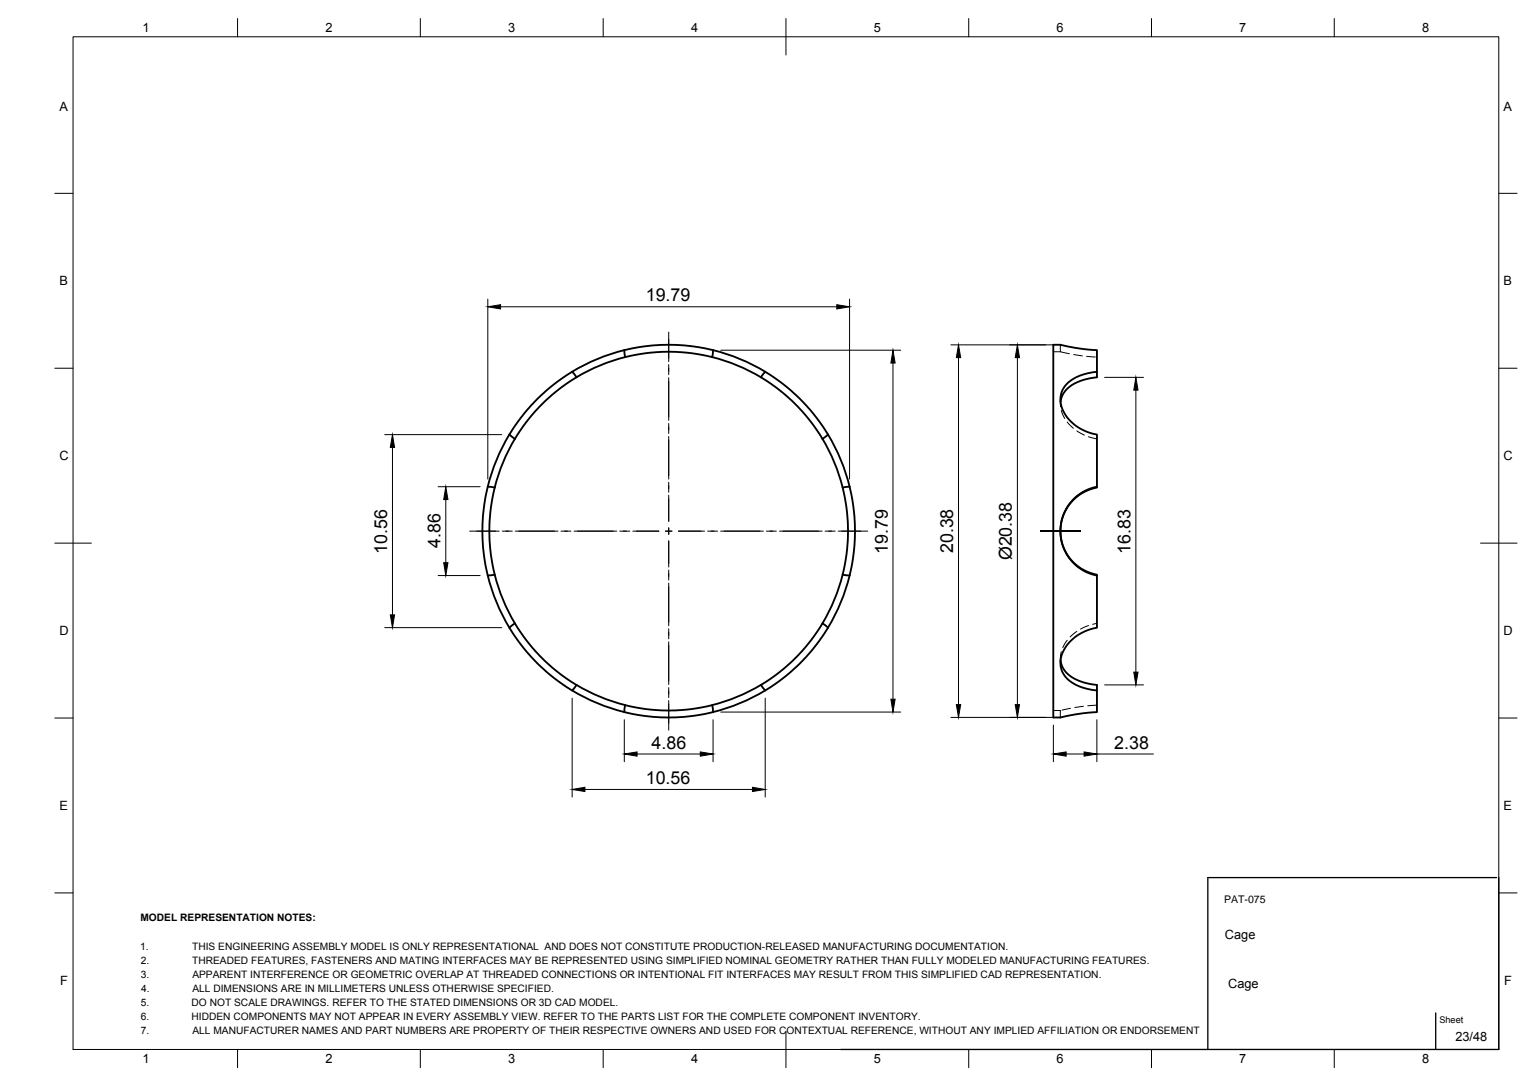
ISO-10303-21;
HEADER;
/* Generated by software containing ST-Developer
 * from STEP Tools, Inc. (www.steptools.com) 
 */

FILE_DESCRIPTION(
/* description */ ('Over-Centre Plunger Toggle Clamp on Slotted Fixture Frame'),
/* implementation_level */ '2;1');

FILE_NAME(
/* name */ 
'Cage.step',
/* time_stamp */ '2026-10-28T03:23:24-07:00',
/* author */ (''),
/* organization */ (''),
/* preprocessor_version */ 'ST-DEVELOPER v20.2',
/* originating_system */ 'Autodesk Translation Framework v15.17.0.0',
/* authorisation */ '');

FILE_SCHEMA (('AUTOMOTIVE_DESIGN { 1 0 10303 214 3 1 1 }'));
ENDSEC;

DATA;
#10=MECHANICAL_DESIGN_GEOMETRIC_PRESENTATION_REPRESENTATION('',(#539),#15212);
#355=B_SPLINE_CURVE_WITH_KNOTS('',3,(#13605,#13606,#13607,#13608,#13609,
#13610,#13611,#13612,#13613,#13614,#13615,#13616,#13617,#13618,#13619,#13620,
#13621,#13622,#13623,#13624,#13625,#13626),.UNSPECIFIED.,.F.,.F.,(4,2,2,
2,2,2,2,2,2,2,4),(0.0473477652366656,0.126350602536658,0.189525903804987,
0.252701205073317,0.313298422430275,0.373895639787233,0.434492857144191,
0.495090074501149,0.558265375769478,0.621440677037807,0.7004435143378),
 .UNSPECIFIED.);
#356=B_SPLINE_CURVE_WITH_KNOTS('',3,(#13630,#13631,#13632,#13633,#13634,
#13635,#13636,#13637,#13638,#13639,#13640,#13641,#13642,#13643,#13644,#13645,
#13646,#13647,#13648,#13649,#13650,#13651),.UNSPECIFIED.,.F.,.F.,(4,2,2,
2,2,2,2,2,2,2,4),(0.0464897534940957,0.0852567806515119,0.170513561303024,
0.246687263103517,0.308657850341199,0.370628437578881,0.432599024816563,
0.494569612054245,0.570743313854739,0.656000094506251,0.694767121663666),
 .UNSPECIFIED.);
#357=B_SPLINE_CURVE_WITH_KNOTS('',3,(#13657,#13658,#13659,#13660,#13661,
#13662,#13663,#13664,#13665,#13666,#13667,#13668,#13669,#13670,#13671,#13672,
#13673,#13674,#13675,#13676,#13677,#13678),.UNSPECIFIED.,.F.,.F.,(4,2,2,
2,2,2,2,2,2,2,4),(0.0464897534940957,0.0852567806515118,0.170513561303024,
0.246687263103517,0.308657850341199,0.370628437578881,0.432599024816563,
0.494569612054245,0.570743313854738,0.65600009450625,0.694767121663666),
 .UNSPECIFIED.);
#358=B_SPLINE_CURVE_WITH_KNOTS('',3,(#13682,#13683,#13684,#13685,#13686,
#13687,#13688,#13689,#13690,#13691,#13692,#13693,#13694,#13695,#13696,#13697,
#13698,#13699,#13700,#13701,#13702,#13703),.UNSPECIFIED.,.F.,.F.,(4,2,2,
2,2,2,2,2,2,2,4),(0.0464897534940957,0.0852567806515119,0.170513561303024,
0.246687263103517,0.308657850341199,0.370628437578881,0.432599024816563,
0.494569612054245,0.570743313854739,0.656000094506251,0.694767121663666),
 .UNSPECIFIED.);
#359=B_SPLINE_CURVE_WITH_KNOTS('',3,(#13707,#13708,#13709,#13710,#13711,
#13712,#13713,#13714,#13715,#13716,#13717,#13718),.UNSPECIFIED.,.F.,.F.,
(4,2,2,2,2,4),(0.0464897534940957,0.0852567806515119,0.170513561303024,
0.246687263103517,0.308657850341199,0.370628437578881),.UNSPECIFIED.);
#360=B_SPLINE_CURVE_WITH_KNOTS('',3,(#13723,#13724,#13725,#13726,#13727,
#13728,#13729,#13730,#13731,#13732,#13733,#13734),.UNSPECIFIED.,.F.,.F.,
(4,2,2,2,2,4),(0.370628437578881,0.432599024816563,0.494569612054245,0.570743313854738,
0.65600009450625,0.694767121663666),.UNSPECIFIED.);
#361=B_SPLINE_CURVE_WITH_KNOTS('',3,(#13738,#13739,#13740,#13741,#13742,
#13743,#13744,#13745,#13746,#13747,#13748,#13749,#13750,#13751,#13752,#13753,
#13754,#13755,#13756,#13757,#13758,#13759),.UNSPECIFIED.,.F.,.F.,(4,2,2,
2,2,2,2,2,2,2,4),(0.0464897534940957,0.0852567806515121,0.170513561303024,
0.246687263103518,0.308657850341199,0.370628437578881,0.432599024816563,
0.494569612054245,0.570743313854738,0.65600009450625,0.694767121663666),
 .UNSPECIFIED.);
#362=B_SPLINE_CURVE_WITH_KNOTS('',3,(#13763,#13764,#13765,#13766,#13767,
#13768,#13769,#13770,#13771,#13772,#13773,#13774,#13775,#13776,#13777,#13778,
#13779,#13780,#13781,#13782,#13783,#13784),.UNSPECIFIED.,.F.,.F.,(4,2,2,
2,2,2,2,2,2,2,4),(0.0464897534940957,0.0852567806515119,0.170513561303024,
0.246687263103517,0.308657850341199,0.370628437578881,0.432599024816563,
0.494569612054245,0.570743313854738,0.65600009450625,0.694767121663667),
 .UNSPECIFIED.);
#363=B_SPLINE_CURVE_WITH_KNOTS('',3,(#13788,#13789,#13790,#13791,#13792,
#13793,#13794,#13795,#13796,#13797,#13798,#13799,#13800,#13801,#13802,#13803,
#13804,#13805,#13806,#13807,#13808,#13809),.UNSPECIFIED.,.F.,.F.,(4,2,2,
2,2,2,2,2,2,2,4),(0.0464897534940957,0.0852567806515119,0.170513561303024,
0.246687263103517,0.308657850341199,0.370628437578881,0.432599024816563,
0.494569612054245,0.570743313854738,0.65600009450625,0.694767121663666),
 .UNSPECIFIED.);
#364=B_SPLINE_CURVE_WITH_KNOTS('',3,(#13813,#13814,#13815,#13816,#13817,
#13818,#13819,#13820,#13821,#13822,#13823,#13824,#13825,#13826,#13827,#13828,
#13829,#13830,#13831,#13832,#13833,#13834),.UNSPECIFIED.,.F.,.F.,(4,2,2,
2,2,2,2,2,2,2,4),(0.0464897534940957,0.0852567806515119,0.170513561303024,
0.246687263103517,0.308657850341199,0.370628437578881,0.432599024816563,
0.494569612054245,0.570743313854739,0.656000094506251,0.694767121663667),
 .UNSPECIFIED.);
#365=B_SPLINE_CURVE_WITH_KNOTS('',3,(#13842,#13843,#13844,#13845,#13846,
#13847,#13848,#13849,#13850,#13851,#13852,#13853,#13854,#13855,#13856,#13857,
#13858,#13859,#13860,#13861,#13862,#13863),.UNSPECIFIED.,.F.,.F.,(4,2,2,
2,2,2,2,2,2,2,4),(0.0473477652366656,0.126350602536658,0.189525903804987,
0.252701205073316,0.313298422430274,0.373895639787232,0.434492857144191,
0.495090074501149,0.558265375769478,0.621440677037807,0.7004435143378),
 .UNSPECIFIED.);
#366=B_SPLINE_CURVE_WITH_KNOTS('',3,(#13871,#13872,#13873,#13874,#13875,
#13876,#13877,#13878,#13879,#13880,#13881,#13882,#13883,#13884,#13885,#13886,
#13887,#13888,#13889,#13890,#13891,#13892),.UNSPECIFIED.,.F.,.F.,(4,2,2,
2,2,2,2,2,2,2,4),(0.0473477652366656,0.126350602536658,0.189525903804987,
0.252701205073317,0.313298422430275,0.373895639787233,0.434492857144191,
0.495090074501149,0.558265375769478,0.621440677037807,0.7004435143378),
 .UNSPECIFIED.);
#367=B_SPLINE_CURVE_WITH_KNOTS('',3,(#13901,#13902,#13903,#13904,#13905,
#13906,#13907,#13908,#13909,#13910,#13911,#13912),.UNSPECIFIED.,.F.,.F.,
(4,2,2,2,2,4),(0.0473477652366656,0.126350602536658,0.189525903804987,0.252701205073316,
0.313298422430275,0.373895639787233),.UNSPECIFIED.);
#368=B_SPLINE_CURVE_WITH_KNOTS('',3,(#13914,#13915,#13916,#13917,#13918,
#13919,#13920,#13921,#13922,#13923,#13924,#13925),.UNSPECIFIED.,.F.,.F.,
(4,2,2,2,2,4),(0.373895639787233,0.434492857144191,0.495090074501149,0.558265375769478,
0.621440677037807,0.7004435143378),.UNSPECIFIED.);
#369=B_SPLINE_CURVE_WITH_KNOTS('',3,(#13932,#13933,#13934,#13935,#13936,
#13937,#13938,#13939,#13940,#13941,#13942,#13943,#13944,#13945,#13946,#13947,
#13948,#13949,#13950,#13951,#13952,#13953),.UNSPECIFIED.,.F.,.F.,(4,2,2,
2,2,2,2,2,2,2,4),(0.0473477652366656,0.126350602536658,0.189525903804987,
0.252701205073316,0.313298422430275,0.373895639787233,0.434492857144191,
0.495090074501149,0.558265375769478,0.621440677037807,0.7004435143378),
 .UNSPECIFIED.);
#370=B_SPLINE_CURVE_WITH_KNOTS('',3,(#13961,#13962,#13963,#13964,#13965,
#13966,#13967,#13968,#13969,#13970,#13971,#13972,#13973,#13974,#13975,#13976,
#13977,#13978,#13979,#13980,#13981,#13982),.UNSPECIFIED.,.F.,.F.,(4,2,2,
2,2,2,2,2,2,2,4),(0.0473477652366656,0.126350602536658,0.189525903804987,
0.252701205073317,0.313298422430275,0.373895639787233,0.434492857144191,
0.495090074501149,0.558265375769478,0.621440677037807,0.7004435143378),
 .UNSPECIFIED.);
#371=B_SPLINE_CURVE_WITH_KNOTS('',3,(#13990,#13991,#13992,#13993,#13994,
#13995,#13996,#13997,#13998,#13999,#14000,#14001,#14002,#14003,#14004,#14005,
#14006,#14007,#14008,#14009,#14010,#14011),.UNSPECIFIED.,.F.,.F.,(4,2,2,
2,2,2,2,2,2,2,4),(0.0473477652366656,0.126350602536658,0.189525903804987,
0.252701205073316,0.313298422430275,0.373895639787233,0.434492857144191,
0.495090074501149,0.558265375769478,0.621440677037807,0.7004435143378),
 .UNSPECIFIED.);
#372=B_SPLINE_CURVE_WITH_KNOTS('',3,(#14020,#14021,#14022,#14023,#14024,
#14025,#14026,#14027,#14028,#14029,#14030,#14031,#14032,#14033,#14034,#14035,
#14036,#14037,#14038,#14039,#14040,#14041),.UNSPECIFIED.,.F.,.F.,(4,2,2,
2,2,2,2,2,2,2,4),(0.0473477652366656,0.126350602536658,0.189525903804987,
0.252701205073317,0.313298422430275,0.373895639787233,0.434492857144191,
0.495090074501149,0.558265375769478,0.621440677037807,0.7004435143378),
 .UNSPECIFIED.);
#387=SPHERICAL_SURFACE('',#9223,0.247676);
#388=SPHERICAL_SURFACE('',#9239,0.247676);
#389=SPHERICAL_SURFACE('',#9244,0.247676);
#390=SPHERICAL_SURFACE('',#9249,0.247676);
#391=SPHERICAL_SURFACE('',#9254,0.247676);
#392=SPHERICAL_SURFACE('',#9259,0.247676);
#393=SPHERICAL_SURFACE('',#9264,0.247676);
#394=SPHERICAL_SURFACE('',#9272,0.247676);
#448=SHAPE_REPRESENTATION_RELATIONSHIP('SRR','None',#15423,#490);
#490=ADVANCED_BREP_SHAPE_REPRESENTATION('',(#589),#15185);
#539=STYLED_ITEM('',(#15719),#589);
#589=MANIFOLD_SOLID_BREP('Continuous crown cage',#8272);
#724=FACE_BOUND('',#1959,.T.);
#942=PLANE('',#9236);
#943=PLANE('',#9241);
#944=PLANE('',#9246);
#945=PLANE('',#9251);
#946=PLANE('',#9256);
#947=PLANE('',#9261);
#948=PLANE('',#9270);
#949=PLANE('',#9274);
#950=PLANE('',#9275);
#1342=FACE_OUTER_BOUND('',#1941,.T.);
#1343=FACE_OUTER_BOUND('',#1942,.T.);
#1344=FACE_OUTER_BOUND('',#1943,.T.);
#1345=FACE_OUTER_BOUND('',#1944,.T.);
#1346=FACE_OUTER_BOUND('',#1945,.T.);
#1347=FACE_OUTER_BOUND('',#1946,.T.);
#1348=FACE_OUTER_BOUND('',#1947,.T.);
#1349=FACE_OUTER_BOUND('',#1948,.T.);
#1350=FACE_OUTER_BOUND('',#1949,.T.);
#1351=FACE_OUTER_BOUND('',#1950,.T.);
#1352=FACE_OUTER_BOUND('',#1951,.T.);
#1353=FACE_OUTER_BOUND('',#1952,.T.);
#1354=FACE_OUTER_BOUND('',#1953,.T.);
#1355=FACE_OUTER_BOUND('',#1954,.T.);
#1356=FACE_OUTER_BOUND('',#1955,.T.);
#1357=FACE_OUTER_BOUND('',#1956,.T.);
#1358=FACE_OUTER_BOUND('',#1957,.T.);
#1359=FACE_OUTER_BOUND('',#1958,.T.);
#1360=FACE_OUTER_BOUND('',#1960,.T.);
#1941=EDGE_LOOP('',(#6709,#6710,#6711,#6712));
#1942=EDGE_LOOP('',(#6713,#6714,#6715,#6716,#6717,#6718,#6719,#6720,#6721,
#6722,#6723,#6724,#6725,#6726,#6727,#6728,#6729,#6730,#6731,#6732));
#1943=EDGE_LOOP('',(#6733,#6734,#6735,#6736));
#1944=EDGE_LOOP('',(#6737,#6738,#6739,#6740));
#1945=EDGE_LOOP('',(#6741,#6742,#6743,#6744));
#1946=EDGE_LOOP('',(#6745,#6746,#6747,#6748));
#1947=EDGE_LOOP('',(#6749,#6750,#6751,#6752));
#1948=EDGE_LOOP('',(#6753,#6754,#6755,#6756,#6757,#6758));
#1949=EDGE_LOOP('',(#6759,#6760,#6761,#6762));
#1950=EDGE_LOOP('',(#6763,#6764,#6765,#6766));
#1951=EDGE_LOOP('',(#6767,#6768,#6769,#6770));
#1952=EDGE_LOOP('',(#6771,#6772,#6773,#6774));
#1953=EDGE_LOOP('',(#6775,#6776,#6777,#6778));
#1954=EDGE_LOOP('',(#6779,#6780,#6781,#6782));
#1955=EDGE_LOOP('',(#6783,#6784,#6785,#6786,#6787,#6788,#6789,#6790,#6791,
#6792,#6793,#6794,#6795,#6796,#6797,#6798,#6799,#6800,#6801,#6802));
#1956=EDGE_LOOP('',(#6803,#6804,#6805,#6806));
#1957=EDGE_LOOP('',(#6807,#6808,#6809,#6810));
#1958=EDGE_LOOP('',(#6811));
#1959=EDGE_LOOP('',(#6812));
#1960=EDGE_LOOP('',(#6813,#6814,#6815,#6816));
#2619=LINE('',#13720,#3249);
#2620=LINE('',#14016,#3250);
#3249=VECTOR('',#11076,1.019052);
#3250=VECTOR('',#11153,0.980948);
#3671=CIRCLE('',#9224,0.243053047864041);
#3672=CIRCLE('',#9225,0.243053047864041);
#3673=CIRCLE('',#9227,1.019052);
#3674=CIRCLE('',#9228,1.019052);
#3675=CIRCLE('',#9229,1.019052);
#3676=CIRCLE('',#9230,1.019052);
#3677=CIRCLE('',#9231,1.019052);
#3678=CIRCLE('',#9232,1.019052);
#3679=CIRCLE('',#9233,1.019052);
#3680=CIRCLE('',#9234,1.019052);
#3681=CIRCLE('',#9235,1.019052);
#3682=CIRCLE('',#9237,0.980948);
#3683=CIRCLE('',#9238,0.243053047864041);
#3684=CIRCLE('',#9240,0.243053047864041);
#3685=CIRCLE('',#9242,0.980948);
#3686=CIRCLE('',#9243,0.243053047864041);
#3687=CIRCLE('',#9245,0.243053047864041);
#3688=CIRCLE('',#9247,0.980948);
#3689=CIRCLE('',#9248,0.243053047864041);
#3690=CIRCLE('',#9250,0.243053047864041);
#3691=CIRCLE('',#9252,0.980948);
#3692=CIRCLE('',#9253,0.243053047864041);
#3693=CIRCLE('',#9255,0.243053047864041);
#3694=CIRCLE('',#9257,0.980948);
#3695=CIRCLE('',#9258,0.243053047864041);
#3696=CIRCLE('',#9260,0.243053047864041);
#3697=CIRCLE('',#9262,0.980948);
#3698=CIRCLE('',#9263,0.243053047864041);
#3699=CIRCLE('',#9265,0.243053047864041);
#3700=CIRCLE('',#9267,0.980948);
#3701=CIRCLE('',#9268,0.980948);
#3702=CIRCLE('',#9269,0.980948);
#3703=CIRCLE('',#9271,0.243053047864041);
#3704=CIRCLE('',#9273,0.243053047864041);
#4247=VERTEX_POINT('',#13603);
#4248=VERTEX_POINT('',#13604);
#4249=VERTEX_POINT('',#13627);
#4250=VERTEX_POINT('',#13629);
#4251=VERTEX_POINT('',#13654);
#4252=VERTEX_POINT('',#13656);
#4253=VERTEX_POINT('',#13679);
#4254=VERTEX_POINT('',#13681);
#4255=VERTEX_POINT('',#13704);
#4256=VERTEX_POINT('',#13706);
#4257=VERTEX_POINT('',#13719);
#4258=VERTEX_POINT('',#13722);
#4259=VERTEX_POINT('',#13735);
#4260=VERTEX_POINT('',#13737);
#4261=VERTEX_POINT('',#13760);
#4262=VERTEX_POINT('',#13762);
#4263=VERTEX_POINT('',#13785);
#4264=VERTEX_POINT('',#13787);
#4265=VERTEX_POINT('',#13810);
#4266=VERTEX_POINT('',#13812);
#4267=VERTEX_POINT('',#13837);
#4268=VERTEX_POINT('',#13841);
#4269=VERTEX_POINT('',#13866);
#4270=VERTEX_POINT('',#13870);
#4271=VERTEX_POINT('',#13895);
#4272=VERTEX_POINT('',#13899);
#4273=VERTEX_POINT('',#13900);
#4274=VERTEX_POINT('',#13927);
#4275=VERTEX_POINT('',#13931);
#4276=VERTEX_POINT('',#13956);
#4277=VERTEX_POINT('',#13960);
#4278=VERTEX_POINT('',#13985);
#4279=VERTEX_POINT('',#13989);
#4280=VERTEX_POINT('',#14014);
#4281=VERTEX_POINT('',#14017);
#4282=VERTEX_POINT('',#14019);
#5115=EDGE_CURVE('',#4247,#4248,#355,.T.);
#5116=EDGE_CURVE('',#4249,#4247,#3671,.T.);
#5117=EDGE_CURVE('',#4250,#4249,#356,.T.);
#5118=EDGE_CURVE('',#4248,#4250,#3672,.T.);
#5119=EDGE_CURVE('',#4251,#4249,#3673,.T.);
#5120=EDGE_CURVE('',#4251,#4252,#357,.T.);
#5121=EDGE_CURVE('',#4253,#4252,#3674,.T.);
#5122=EDGE_CURVE('',#4253,#4254,#358,.T.);
#5123=EDGE_CURVE('',#4255,#4254,#3675,.T.);
#5124=EDGE_CURVE('',#4255,#4256,#359,.T.);
#5125=EDGE_CURVE('',#4256,#4257,#2619,.T.);
#5126=EDGE_CURVE('',#4257,#4257,#3676,.T.);
#5127=EDGE_CURVE('',#4256,#4258,#360,.T.);
#5128=EDGE_CURVE('',#4259,#4258,#3677,.T.);
#5129=EDGE_CURVE('',#4259,#4260,#361,.T.);
#5130=EDGE_CURVE('',#4261,#4260,#3678,.T.);
#5131=EDGE_CURVE('',#4261,#4262,#362,.T.);
#5132=EDGE_CURVE('',#4263,#4262,#3679,.T.);
#5133=EDGE_CURVE('',#4263,#4264,#363,.T.);
#5134=EDGE_CURVE('',#4265,#4264,#3680,.T.);
#5135=EDGE_CURVE('',#4265,#4266,#364,.T.);
#5136=EDGE_CURVE('',#4250,#4266,#3681,.T.);
#5137=EDGE_CURVE('',#4247,#4267,#3682,.T.);
#5138=EDGE_CURVE('',#4267,#4251,#3683,.T.);
#5139=EDGE_CURVE('',#4268,#4267,#365,.T.);
#5140=EDGE_CURVE('',#4252,#4268,#3684,.T.);
#5141=EDGE_CURVE('',#4268,#4269,#3685,.T.);
#5142=EDGE_CURVE('',#4269,#4253,#3686,.T.);
#5143=EDGE_CURVE('',#4270,#4269,#366,.T.);
#5144=EDGE_CURVE('',#4254,#4270,#3687,.T.);
#5145=EDGE_CURVE('',#4270,#4271,#3688,.T.);
#5146=EDGE_CURVE('',#4271,#4255,#3689,.T.);
#5147=EDGE_CURVE('',#4272,#4273,#367,.T.);
#5148=EDGE_CURVE('',#4258,#4272,#3690,.T.);
#5149=EDGE_CURVE('',#4273,#4271,#368,.T.);
#5150=EDGE_CURVE('',#4272,#4274,#3691,.T.);
#5151=EDGE_CURVE('',#4274,#4259,#3692,.T.);
#5152=EDGE_CURVE('',#4275,#4274,#369,.T.);
#5153=EDGE_CURVE('',#4260,#4275,#3693,.T.);
#5154=EDGE_CURVE('',#4275,#4276,#3694,.T.);
#5155=EDGE_CURVE('',#4276,#4261,#3695,.T.);
#5156=EDGE_CURVE('',#4277,#4276,#370,.T.);
#5157=EDGE_CURVE('',#4262,#4277,#3696,.T.);
#5158=EDGE_CURVE('',#4277,#4278,#3697,.T.);
#5159=EDGE_CURVE('',#4278,#4263,#3698,.T.);
#5160=EDGE_CURVE('',#4279,#4278,#371,.T.);
#5161=EDGE_CURVE('',#4264,#4279,#3699,.T.);
#5162=EDGE_CURVE('',#4280,#4280,#3700,.T.);
#5163=EDGE_CURVE('',#4280,#4273,#2620,.T.);
#5164=EDGE_CURVE('',#4281,#4248,#3701,.T.);
#5165=EDGE_CURVE('',#4281,#4282,#372,.T.);
#5166=EDGE_CURVE('',#4279,#4282,#3702,.T.);
#5167=EDGE_CURVE('',#4266,#4281,#3703,.T.);
#5168=EDGE_CURVE('',#4282,#4265,#3704,.T.);
#6709=ORIENTED_EDGE('',*,*,#5115,.F.);
#6710=ORIENTED_EDGE('',*,*,#5116,.F.);
#6711=ORIENTED_EDGE('',*,*,#5117,.F.);
#6712=ORIENTED_EDGE('',*,*,#5118,.F.);
#6713=ORIENTED_EDGE('',*,*,#5117,.T.);
#6714=ORIENTED_EDGE('',*,*,#5119,.F.);
#6715=ORIENTED_EDGE('',*,*,#5120,.T.);
#6716=ORIENTED_EDGE('',*,*,#5121,.F.);
#6717=ORIENTED_EDGE('',*,*,#5122,.T.);
#6718=ORIENTED_EDGE('',*,*,#5123,.F.);
#6719=ORIENTED_EDGE('',*,*,#5124,.T.);
#6720=ORIENTED_EDGE('',*,*,#5125,.T.);
#6721=ORIENTED_EDGE('',*,*,#5126,.F.);
#6722=ORIENTED_EDGE('',*,*,#5125,.F.);
#6723=ORIENTED_EDGE('',*,*,#5127,.T.);
#6724=ORIENTED_EDGE('',*,*,#5128,.F.);
#6725=ORIENTED_EDGE('',*,*,#5129,.T.);
#6726=ORIENTED_EDGE('',*,*,#5130,.F.);
#6727=ORIENTED_EDGE('',*,*,#5131,.T.);
#6728=ORIENTED_EDGE('',*,*,#5132,.F.);
#6729=ORIENTED_EDGE('',*,*,#5133,.T.);
#6730=ORIENTED_EDGE('',*,*,#5134,.F.);
#6731=ORIENTED_EDGE('',*,*,#5135,.T.);
#6732=ORIENTED_EDGE('',*,*,#5136,.F.);
#6733=ORIENTED_EDGE('',*,*,#5116,.T.);
#6734=ORIENTED_EDGE('',*,*,#5137,.T.);
#6735=ORIENTED_EDGE('',*,*,#5138,.T.);
#6736=ORIENTED_EDGE('',*,*,#5119,.T.);
#6737=ORIENTED_EDGE('',*,*,#5139,.F.);
#6738=ORIENTED_EDGE('',*,*,#5140,.F.);
#6739=ORIENTED_EDGE('',*,*,#5120,.F.);
#6740=ORIENTED_EDGE('',*,*,#5138,.F.);
#6741=ORIENTED_EDGE('',*,*,#5140,.T.);
#6742=ORIENTED_EDGE('',*,*,#5141,.T.);
#6743=ORIENTED_EDGE('',*,*,#5142,.T.);
#6744=ORIENTED_EDGE('',*,*,#5121,.T.);
#6745=ORIENTED_EDGE('',*,*,#5143,.F.);
#6746=ORIENTED_EDGE('',*,*,#5144,.F.);
#6747=ORIENTED_EDGE('',*,*,#5122,.F.);
#6748=ORIENTED_EDGE('',*,*,#5142,.F.);
#6749=ORIENTED_EDGE('',*,*,#5144,.T.);
#6750=ORIENTED_EDGE('',*,*,#5145,.T.);
#6751=ORIENTED_EDGE('',*,*,#5146,.T.);
#6752=ORIENTED_EDGE('',*,*,#5123,.T.);
#6753=ORIENTED_EDGE('',*,*,#5147,.F.);
#6754=ORIENTED_EDGE('',*,*,#5148,.F.);
#6755=ORIENTED_EDGE('',*,*,#5127,.F.);
#6756=ORIENTED_EDGE('',*,*,#5124,.F.);
#6757=ORIENTED_EDGE('',*,*,#5146,.F.);
#6758=ORIENTED_EDGE('',*,*,#5149,.F.);
#6759=ORIENTED_EDGE('',*,*,#5148,.T.);
#6760=ORIENTED_EDGE('',*,*,#5150,.T.);
#6761=ORIENTED_EDGE('',*,*,#5151,.T.);
#6762=ORIENTED_EDGE('',*,*,#5128,.T.);
#6763=ORIENTED_EDGE('',*,*,#5152,.F.);
#6764=ORIENTED_EDGE('',*,*,#5153,.F.);
#6765=ORIENTED_EDGE('',*,*,#5129,.F.);
#6766=ORIENTED_EDGE('',*,*,#5151,.F.);
#6767=ORIENTED_EDGE('',*,*,#5153,.T.);
#6768=ORIENTED_EDGE('',*,*,#5154,.T.);
#6769=ORIENTED_EDGE('',*,*,#5155,.T.);
#6770=ORIENTED_EDGE('',*,*,#5130,.T.);
#6771=ORIENTED_EDGE('',*,*,#5156,.F.);
#6772=ORIENTED_EDGE('',*,*,#5157,.F.);
#6773=ORIENTED_EDGE('',*,*,#5131,.F.);
#6774=ORIENTED_EDGE('',*,*,#5155,.F.);
#6775=ORIENTED_EDGE('',*,*,#5157,.T.);
#6776=ORIENTED_EDGE('',*,*,#5158,.T.);
#6777=ORIENTED_EDGE('',*,*,#5159,.T.);
#6778=ORIENTED_EDGE('',*,*,#5132,.T.);
#6779=ORIENTED_EDGE('',*,*,#5133,.F.);
#6780=ORIENTED_EDGE('',*,*,#5159,.F.);
#6781=ORIENTED_EDGE('',*,*,#5160,.F.);
#6782=ORIENTED_EDGE('',*,*,#5161,.F.);
#6783=ORIENTED_EDGE('',*,*,#5162,.F.);
#6784=ORIENTED_EDGE('',*,*,#5163,.T.);
#6785=ORIENTED_EDGE('',*,*,#5149,.T.);
#6786=ORIENTED_EDGE('',*,*,#5145,.F.);
#6787=ORIENTED_EDGE('',*,*,#5143,.T.);
#6788=ORIENTED_EDGE('',*,*,#5141,.F.);
#6789=ORIENTED_EDGE('',*,*,#5139,.T.);
#6790=ORIENTED_EDGE('',*,*,#5137,.F.);
#6791=ORIENTED_EDGE('',*,*,#5115,.T.);
#6792=ORIENTED_EDGE('',*,*,#5164,.F.);
#6793=ORIENTED_EDGE('',*,*,#5165,.T.);
#6794=ORIENTED_EDGE('',*,*,#5166,.F.);
#6795=ORIENTED_EDGE('',*,*,#5160,.T.);
#6796=ORIENTED_EDGE('',*,*,#5158,.F.);
#6797=ORIENTED_EDGE('',*,*,#5156,.T.);
#6798=ORIENTED_EDGE('',*,*,#5154,.F.);
#6799=ORIENTED_EDGE('',*,*,#5152,.T.);
#6800=ORIENTED_EDGE('',*,*,#5150,.F.);
#6801=ORIENTED_EDGE('',*,*,#5147,.T.);
#6802=ORIENTED_EDGE('',*,*,#5163,.F.);
#6803=ORIENTED_EDGE('',*,*,#5118,.T.);
#6804=ORIENTED_EDGE('',*,*,#5136,.T.);
#6805=ORIENTED_EDGE('',*,*,#5167,.T.);
#6806=ORIENTED_EDGE('',*,*,#5164,.T.);
#6807=ORIENTED_EDGE('',*,*,#5135,.F.);
#6808=ORIENTED_EDGE('',*,*,#5168,.F.);
#6809=ORIENTED_EDGE('',*,*,#5165,.F.);
#6810=ORIENTED_EDGE('',*,*,#5167,.F.);
#6811=ORIENTED_EDGE('',*,*,#5126,.T.);
#6812=ORIENTED_EDGE('',*,*,#5162,.T.);
#6813=ORIENTED_EDGE('',*,*,#5161,.T.);
#6814=ORIENTED_EDGE('',*,*,#5166,.T.);
#6815=ORIENTED_EDGE('',*,*,#5168,.T.);
#6816=ORIENTED_EDGE('',*,*,#5134,.T.);
#7695=CYLINDRICAL_SURFACE('',#9226,1.019052);
#7696=CYLINDRICAL_SURFACE('',#9266,0.980948);
#8014=ADVANCED_FACE('',(#1342),#387,.F.);
#8015=ADVANCED_FACE('',(#1343),#7695,.T.);
#8016=ADVANCED_FACE('',(#1344),#942,.T.);
#8017=ADVANCED_FACE('',(#1345),#388,.F.);
#8018=ADVANCED_FACE('',(#1346),#943,.T.);
#8019=ADVANCED_FACE('',(#1347),#389,.F.);
#8020=ADVANCED_FACE('',(#1348),#944,.T.);
#8021=ADVANCED_FACE('',(#1349),#390,.F.);
#8022=ADVANCED_FACE('',(#1350),#945,.T.);
#8023=ADVANCED_FACE('',(#1351),#391,.F.);
#8024=ADVANCED_FACE('',(#1352),#946,.T.);
#8025=ADVANCED_FACE('',(#1353),#392,.F.);
#8026=ADVANCED_FACE('',(#1354),#947,.T.);
#8027=ADVANCED_FACE('',(#1355),#393,.F.);
#8028=ADVANCED_FACE('',(#1356),#7696,.F.);
#8029=ADVANCED_FACE('',(#1357),#948,.T.);
#8030=ADVANCED_FACE('',(#1358),#394,.F.);
#8031=ADVANCED_FACE('',(#1359,#724),#949,.T.);
#8032=ADVANCED_FACE('',(#1360),#950,.T.);
#8272=CLOSED_SHELL('',(#8014,#8015,#8016,#8017,#8018,#8019,#8020,#8021,
#8022,#8023,#8024,#8025,#8026,#8027,#8028,#8029,#8030,#8031,#8032));
#9222=AXIS2_PLACEMENT_3D('',#13601,#11060,#11061);
#9223=AXIS2_PLACEMENT_3D('',#13602,#11062,#11063);
#9224=AXIS2_PLACEMENT_3D('',#13628,#11064,#11065);
#9225=AXIS2_PLACEMENT_3D('',#13652,#11066,#11067);
#9226=AXIS2_PLACEMENT_3D('',#13653,#11068,#11069);
#9227=AXIS2_PLACEMENT_3D('',#13655,#11070,#11071);
#9228=AXIS2_PLACEMENT_3D('',#13680,#11072,#11073);
#9229=AXIS2_PLACEMENT_3D('',#13705,#11074,#11075);
#9230=AXIS2_PLACEMENT_3D('',#13721,#11077,#11078);
#9231=AXIS2_PLACEMENT_3D('',#13736,#11079,#11080);
#9232=AXIS2_PLACEMENT_3D('',#13761,#11081,#11082);
#9233=AXIS2_PLACEMENT_3D('',#13786,#11083,#11084);
#9234=AXIS2_PLACEMENT_3D('',#13811,#11085,#11086);
#9235=AXIS2_PLACEMENT_3D('',#13835,#11087,#11088);
#9236=AXIS2_PLACEMENT_3D('',#13836,#11089,#11090);
#9237=AXIS2_PLACEMENT_3D('',#13838,#11091,#11092);
#9238=AXIS2_PLACEMENT_3D('',#13839,#11093,#11094);
#9239=AXIS2_PLACEMENT_3D('',#13840,#11095,#11096);
#9240=AXIS2_PLACEMENT_3D('',#13864,#11097,#11098);
#9241=AXIS2_PLACEMENT_3D('',#13865,#11099,#11100);
#9242=AXIS2_PLACEMENT_3D('',#13867,#11101,#11102);
#9243=AXIS2_PLACEMENT_3D('',#13868,#11103,#11104);
#9244=AXIS2_PLACEMENT_3D('',#13869,#11105,#11106);
#9245=AXIS2_PLACEMENT_3D('',#13893,#11107,#11108);
#9246=AXIS2_PLACEMENT_3D('',#13894,#11109,#11110);
#9247=AXIS2_PLACEMENT_3D('',#13896,#11111,#11112);
#9248=AXIS2_PLACEMENT_3D('',#13897,#11113,#11114);
#9249=AXIS2_PLACEMENT_3D('',#13898,#11115,#11116);
#9250=AXIS2_PLACEMENT_3D('',#13913,#11117,#11118);
#9251=AXIS2_PLACEMENT_3D('',#13926,#11119,#11120);
#9252=AXIS2_PLACEMENT_3D('',#13928,#11121,#11122);
#9253=AXIS2_PLACEMENT_3D('',#13929,#11123,#11124);
#9254=AXIS2_PLACEMENT_3D('',#13930,#11125,#11126);
#9255=AXIS2_PLACEMENT_3D('',#13954,#11127,#11128);
#9256=AXIS2_PLACEMENT_3D('',#13955,#11129,#11130);
#9257=AXIS2_PLACEMENT_3D('',#13957,#11131,#11132);
#9258=AXIS2_PLACEMENT_3D('',#13958,#11133,#11134);
#9259=AXIS2_PLACEMENT_3D('',#13959,#11135,#11136);
#9260=AXIS2_PLACEMENT_3D('',#13983,#11137,#11138);
#9261=AXIS2_PLACEMENT_3D('',#13984,#11139,#11140);
#9262=AXIS2_PLACEMENT_3D('',#13986,#11141,#11142);
#9263=AXIS2_PLACEMENT_3D('',#13987,#11143,#11144);
#9264=AXIS2_PLACEMENT_3D('',#13988,#11145,#11146);
#9265=AXIS2_PLACEMENT_3D('',#14012,#11147,#11148);
#9266=AXIS2_PLACEMENT_3D('',#14013,#11149,#11150);
#9267=AXIS2_PLACEMENT_3D('',#14015,#11151,#11152);
#9268=AXIS2_PLACEMENT_3D('',#14018,#11154,#11155);
#9269=AXIS2_PLACEMENT_3D('',#14042,#11156,#11157);
#9270=AXIS2_PLACEMENT_3D('',#14043,#11158,#11159);
#9271=AXIS2_PLACEMENT_3D('',#14044,#11160,#11161);
#9272=AXIS2_PLACEMENT_3D('',#14045,#11162,#11163);
#9273=AXIS2_PLACEMENT_3D('',#14046,#11164,#11165);
#9274=AXIS2_PLACEMENT_3D('',#14047,#11166,#11167);
#9275=AXIS2_PLACEMENT_3D('',#14048,#11168,#11169);
#11060=DIRECTION('axis',(0.,0.,1.));
#11061=DIRECTION('refdir',(1.,0.,0.));
#11062=DIRECTION('center_axis',(0.,0.,1.));
#11063=DIRECTION('ref_axis',(1.,0.,0.));
#11064=DIRECTION('center_axis',(0.,-1.,0.));
#11065=DIRECTION('ref_axis',(0.,0.,-1.));
#11066=DIRECTION('center_axis',(0.,-1.,0.));
#11067=DIRECTION('ref_axis',(0.,0.,-1.));
#11068=DIRECTION('center_axis',(0.,1.,0.));
#11069=DIRECTION('ref_axis',(1.,0.,0.));
#11070=DIRECTION('center_axis',(0.,1.,0.));
#11071=DIRECTION('ref_axis',(1.,0.,0.));
#11072=DIRECTION('center_axis',(0.,1.,0.));
#11073=DIRECTION('ref_axis',(1.,0.,0.));
#11074=DIRECTION('center_axis',(0.,1.,0.));
#11075=DIRECTION('ref_axis',(1.,0.,0.));
#11076=DIRECTION('',(0.,-1.,0.));
#11077=DIRECTION('center_axis',(0.,-1.,0.));
#11078=DIRECTION('ref_axis',(1.,0.,0.));
#11079=DIRECTION('center_axis',(0.,1.,0.));
#11080=DIRECTION('ref_axis',(1.,0.,0.));
#11081=DIRECTION('center_axis',(0.,1.,0.));
#11082=DIRECTION('ref_axis',(1.,0.,0.));
#11083=DIRECTION('center_axis',(0.,1.,0.));
#11084=DIRECTION('ref_axis',(1.,0.,0.));
#11085=DIRECTION('center_axis',(0.,1.,0.));
#11086=DIRECTION('ref_axis',(1.,0.,0.));
#11087=DIRECTION('center_axis',(0.,1.,0.));
#11088=DIRECTION('ref_axis',(1.,0.,0.));
#11089=DIRECTION('center_axis',(0.,1.,0.));
#11090=DIRECTION('ref_axis',(1.,0.,0.));
#11091=DIRECTION('center_axis',(0.,-1.,0.));
#11092=DIRECTION('ref_axis',(1.,0.,0.));
#11093=DIRECTION('center_axis',(0.,-1.,0.));
#11094=DIRECTION('ref_axis',(0.,0.,-1.));
#11095=DIRECTION('center_axis',(6.12323399573677E-17,0.,1.));
#11096=DIRECTION('ref_axis',(1.,0.,0.));
#11097=DIRECTION('center_axis',(0.,-1.,0.));
#11098=DIRECTION('ref_axis',(0.,0.,-1.));
#11099=DIRECTION('center_axis',(0.,1.,0.));
#11100=DIRECTION('ref_axis',(1.,0.,0.));
#11101=DIRECTION('center_axis',(0.,-1.,0.));
#11102=DIRECTION('ref_axis',(1.,0.,0.));
#11103=DIRECTION('center_axis',(0.,-1.,0.));
#11104=DIRECTION('ref_axis',(0.,0.,-1.));
#11105=DIRECTION('center_axis',(0.,0.,1.));
#11106=DIRECTION('ref_axis',(1.,0.,0.));
#11107=DIRECTION('center_axis',(0.,-1.,0.));
#11108=DIRECTION('ref_axis',(0.,0.,-1.));
#11109=DIRECTION('center_axis',(0.,1.,0.));
#11110=DIRECTION('ref_axis',(1.,0.,0.));
#11111=DIRECTION('center_axis',(0.,-1.,0.));
#11112=DIRECTION('ref_axis',(1.,0.,0.));
#11113=DIRECTION('center_axis',(0.,-1.,0.));
#11114=DIRECTION('ref_axis',(0.,0.,-1.));
#11115=DIRECTION('center_axis',(0.,0.,1.));
#11116=DIRECTION('ref_axis',(1.,0.,0.));
#11117=DIRECTION('center_axis',(0.,-1.,0.));
#11118=DIRECTION('ref_axis',(0.,0.,-1.));
#11119=DIRECTION('center_axis',(0.,1.,0.));
#11120=DIRECTION('ref_axis',(1.,0.,0.));
#11121=DIRECTION('center_axis',(0.,-1.,0.));
#11122=DIRECTION('ref_axis',(1.,0.,0.));
#11123=DIRECTION('center_axis',(0.,-1.,0.));
#11124=DIRECTION('ref_axis',(0.,0.,-1.));
#11125=DIRECTION('center_axis',(0.,0.,1.));
#11126=DIRECTION('ref_axis',(1.,0.,0.));
#11127=DIRECTION('center_axis',(0.,-1.,0.));
#11128=DIRECTION('ref_axis',(0.,0.,-1.));
#11129=DIRECTION('center_axis',(0.,1.,0.));
#11130=DIRECTION('ref_axis',(1.,0.,0.));
#11131=DIRECTION('center_axis',(0.,-1.,0.));
#11132=DIRECTION('ref_axis',(1.,0.,0.));
#11133=DIRECTION('center_axis',(0.,-1.,0.));
#11134=DIRECTION('ref_axis',(0.,0.,-1.));
#11135=DIRECTION('center_axis',(6.12323399573676E-17,0.,1.));
#11136=DIRECTION('ref_axis',(1.,0.,0.));
#11137=DIRECTION('center_axis',(0.,-1.,0.));
#11138=DIRECTION('ref_axis',(0.,0.,-1.));
#11139=DIRECTION('center_axis',(0.,1.,0.));
#11140=DIRECTION('ref_axis',(1.,0.,0.));
#11141=DIRECTION('center_axis',(0.,-1.,0.));
#11142=DIRECTION('ref_axis',(1.,0.,0.));
#11143=DIRECTION('center_axis',(0.,-1.,0.));
#11144=DIRECTION('ref_axis',(0.,0.,-1.));
#11145=DIRECTION('center_axis',(0.,0.,1.));
#11146=DIRECTION('ref_axis',(1.,0.,0.));
#11147=DIRECTION('center_axis',(0.,-1.,0.));
#11148=DIRECTION('ref_axis',(0.,0.,-1.));
#11149=DIRECTION('center_axis',(0.,1.,0.));
#11150=DIRECTION('ref_axis',(1.,0.,0.));
#11151=DIRECTION('center_axis',(0.,1.,0.));
#11152=DIRECTION('ref_axis',(1.,0.,0.));
#11153=DIRECTION('',(0.,1.,0.));
#11154=DIRECTION('center_axis',(0.,-1.,0.));
#11155=DIRECTION('ref_axis',(1.,0.,0.));
#11156=DIRECTION('center_axis',(0.,-1.,0.));
#11157=DIRECTION('ref_axis',(1.,0.,0.));
#11158=DIRECTION('center_axis',(0.,1.,0.));
#11159=DIRECTION('ref_axis',(1.,0.,0.));
#11160=DIRECTION('center_axis',(0.,-1.,0.));
#11161=DIRECTION('ref_axis',(0.,0.,-1.));
#11162=DIRECTION('center_axis',(0.,0.,1.));
#11163=DIRECTION('ref_axis',(1.,0.,0.));
#11164=DIRECTION('center_axis',(0.,-1.,0.));
#11165=DIRECTION('ref_axis',(0.,0.,-1.));
#11166=DIRECTION('center_axis',(0.,-1.,0.));
#11167=DIRECTION('ref_axis',(-1.,0.,0.));
#11168=DIRECTION('center_axis',(0.,1.,0.));
#11169=DIRECTION('ref_axis',(1.,0.,0.));
#13601=CARTESIAN_POINT('',(0.,0.,0.));
#13602=CARTESIAN_POINT('Origin',(0.707106781186547,0.,0.707106781186548));
#13603=CARTESIAN_POINT('',(0.504455939115715,-0.04763,0.841298510752802));
#13604=CARTESIAN_POINT('',(0.841298510752802,-0.04763,0.504455939115715));
#13605=CARTESIAN_POINT('Ctrl Pts',(0.504455939115715,-0.04763,0.841298510752802));
#13606=CARTESIAN_POINT('Ctrl Pts',(0.508899795931835,-0.0740444353928835,
0.838633903678357));
#13607=CARTESIAN_POINT('Ctrl Pts',(0.517157748491652,-0.0999305678883309,
0.833661031856294));
#13608=CARTESIAN_POINT('Ctrl Pts',(0.537715343527944,-0.142345102874864,
0.820511285096538));
#13609=CARTESIAN_POINT('Ctrl Pts',(0.548874290046456,-0.159766064500479,
0.813159949759));
#13610=CARTESIAN_POINT('Ctrl Pts',(0.573915184558107,-0.190326085855194,
0.795684265985089));
#13611=CARTESIAN_POINT('Ctrl Pts',(0.587792702767295,-0.203463743702801,
0.78555112003688));
#13612=CARTESIAN_POINT('Ctrl Pts',(0.615966552324775,-0.224161999508995,
0.763642258217233));
#13613=CARTESIAN_POINT('Ctrl Pts',(0.631684198665438,-0.232861760990032,
0.750785745543687));
#13614=CARTESIAN_POINT('Ctrl Pts',(0.663382628119203,-0.244251601209411,
0.722929908501543));
#13615=CARTESIAN_POINT('Ctrl Pts',(0.679352081686668,-0.246942143572133,
0.707917883896095));
#13616=CARTESIAN_POINT('Ctrl Pts',(0.707917883896095,-0.246942143572133,
0.679352081686668));
#13617=CARTESIAN_POINT('Ctrl Pts',(0.722929908501543,-0.244251601209411,
0.663382628119203));
#13618=CARTESIAN_POINT('Ctrl Pts',(0.750785745543687,-0.232861760990032,
0.631684198665439));
#13619=CARTESIAN_POINT('Ctrl Pts',(0.763642258217232,-0.224161999508995,
0.615966552324775));
#13620=CARTESIAN_POINT('Ctrl Pts',(0.78555112003688,-0.203463743702801,
0.587792702767295));
#13621=CARTESIAN_POINT('Ctrl Pts',(0.795684265985088,-0.190326085855194,
0.573915184558108));
#13622=CARTESIAN_POINT('Ctrl Pts',(0.813159949759,-0.15976606450048,0.548874290046456));
#13623=CARTESIAN_POINT('Ctrl Pts',(0.820511285096538,-0.142345102874864,
0.537715343527944));
#13624=CARTESIAN_POINT('Ctrl Pts',(0.833661031856294,-0.099930567888331,
0.517157748491653));
#13625=CARTESIAN_POINT('Ctrl Pts',(0.838633903678357,-0.0740444353928835,
0.508899795931835));
#13626=CARTESIAN_POINT('Ctrl Pts',(0.841298510752801,-0.0476299999999999,
0.504455939115715));
#13627=CARTESIAN_POINT('',(0.528110872004958,-0.04763,0.871530771444223));
#13628=CARTESIAN_POINT('Origin',(0.707106781186547,-0.04763,0.707106781186548));
#13629=CARTESIAN_POINT('',(0.871530771444223,-0.04763,0.528110872004959));
#13630=CARTESIAN_POINT('Ctrl Pts',(0.871530771444223,-0.0476300000000001,
0.528110872004958));
#13631=CARTESIAN_POINT('Ctrl Pts',(0.87014664509073,-0.0609922781173483,
0.530395067942936));
#13632=CARTESIAN_POINT('Ctrl Pts',(0.868149331745851,-0.0742967091364493,
0.533674141594226));
#13633=CARTESIAN_POINT('Ctrl Pts',(0.85981294420286,-0.115492077056649,
0.54708917182331));
#13634=CARTESIAN_POINT('Ctrl Pts',(0.850993704737257,-0.141695629206859,
0.560922177770136));
#13635=CARTESIAN_POINT('Ctrl Pts',(0.830754510485543,-0.181890537957859,
0.590422647829571));
#13636=CARTESIAN_POINT('Ctrl Pts',(0.816896541396381,-0.201072148666545,
0.609616703125488));
#13637=CARTESIAN_POINT('Ctrl Pts',(0.792310597819928,-0.223955109275652,
0.641117951819998));
#13638=CARTESIAN_POINT('Ctrl Pts',(0.779109323683612,-0.232742381310829,
0.657208095763053));
#13639=CARTESIAN_POINT('Ctrl Pts',(0.750552691816206,-0.244234834628584,
0.68964083160521));
#13640=CARTESIAN_POINT('Ctrl Pts',(0.735185187071673,-0.246942143572133,
0.705971972091755));
#13641=CARTESIAN_POINT('Ctrl Pts',(0.705971972091754,-0.246942143572133,
0.735185187071673));
#13642=CARTESIAN_POINT('Ctrl Pts',(0.689640831605209,-0.244234834628584,
0.750552691816206));
#13643=CARTESIAN_POINT('Ctrl Pts',(0.657208095763052,-0.232742381310829,
0.779109323683612));
#13644=CARTESIAN_POINT('Ctrl Pts',(0.641117951819998,-0.223955109275652,
0.792310597819928));
#13645=CARTESIAN_POINT('Ctrl Pts',(0.609616703125487,-0.201072148666545,
0.816896541396382));
#13646=CARTESIAN_POINT('Ctrl Pts',(0.590422647829571,-0.181890537957858,
0.830754510485544));
#13647=CARTESIAN_POINT('Ctrl Pts',(0.560922177770135,-0.141695629206858,
0.850993704737257));
#13648=CARTESIAN_POINT('Ctrl Pts',(0.547089171823309,-0.115492077056649,
0.859812944202861));
#13649=CARTESIAN_POINT('Ctrl Pts',(0.533674141594226,-0.0742967091364491,
0.868149331745852));
#13650=CARTESIAN_POINT('Ctrl Pts',(0.530395067942936,-0.0609922781173483,
0.870146645090731));
#13651=CARTESIAN_POINT('Ctrl Pts',(0.528110872004958,-0.0476300000000001,
0.871530771444223));
#13652=CARTESIAN_POINT('Origin',(0.707106781186547,-0.04763,0.707106781186548));
#13653=CARTESIAN_POINT('Origin',(0.,-0.166705,0.));
#13654=CARTESIAN_POINT('',(0.242834539687906,-0.04763,0.989696097314));
#13655=CARTESIAN_POINT('Origin',(0.,-0.04763,0.));
#13656=CARTESIAN_POINT('',(-0.242834539687907,-0.04763,0.989696097314));
#13657=CARTESIAN_POINT('Ctrl Pts',(0.242834539687906,-0.04763,0.989696097314));
#13658=CARTESIAN_POINT('Ctrl Pts',(0.24024064412003,-0.0609922781173483,
0.990332542620729));
#13659=CARTESIAN_POINT('Ctrl Pts',(0.236509675094874,-0.0742967091364492,
0.991238884025248));
#13660=CARTESIAN_POINT('Ctrl Pts',(0.221129100087819,-0.115492077056649,
0.994830026707808));
#13661=CARTESIAN_POINT('Ctrl Pts',(0.205111543747588,-0.141695629206859,
0.998375294985966));
#13662=CARTESIAN_POINT('Ctrl Pts',(0.169940289819232,-0.181890537957859,
1.00492400591205));
#13663=CARTESIAN_POINT('Ctrl Pts',(0.1465689792446,-0.201072148666545,1.00869718865384));
#13664=CARTESIAN_POINT('Ctrl Pts',(0.106909345252087,-0.223955109275652,
1.01358704779679));
#13665=CARTESIAN_POINT('Ctrl Pts',(0.0861971848975941,-0.232742381310829,
1.0156297872271));
#13666=CARTESIAN_POINT('Ctrl Pts',(0.0430711894098822,-0.244234834628584,
1.01837060663223));
#13667=CARTESIAN_POINT('Ctrl Pts',(0.0206568624125605,-0.246942143572133,
1.019052));
#13668=CARTESIAN_POINT('Ctrl Pts',(-0.0206568624125608,-0.246942143572133,
1.019052));
#13669=CARTESIAN_POINT('Ctrl Pts',(-0.0430711894098825,-0.244234834628584,
1.01837060663223));
#13670=CARTESIAN_POINT('Ctrl Pts',(-0.0861971848975943,-0.232742381310829,
1.0156297872271));
#13671=CARTESIAN_POINT('Ctrl Pts',(-0.106909345252088,-0.223955109275652,
1.01358704779679));
#13672=CARTESIAN_POINT('Ctrl Pts',(-0.1465689792446,-0.201072148666545,
1.00869718865384));
#13673=CARTESIAN_POINT('Ctrl Pts',(-0.169940289819232,-0.181890537957859,
1.00492400591205));
#13674=CARTESIAN_POINT('Ctrl Pts',(-0.205111543747588,-0.141695629206859,
0.998375294985966));
#13675=CARTESIAN_POINT('Ctrl Pts',(-0.221129100087819,-0.115492077056649,
0.994830026707808));
#13676=CARTESIAN_POINT('Ctrl Pts',(-0.236509675094875,-0.0742967091364493,
0.991238884025248));
#13677=CARTESIAN_POINT('Ctrl Pts',(-0.24024064412003,-0.0609922781173483,
0.990332542620729));
#13678=CARTESIAN_POINT('Ctrl Pts',(-0.242834539687907,-0.04763,0.989696097314));
#13679=CARTESIAN_POINT('',(-0.528110872004959,-0.04763,0.871530771444223));
#13680=CARTESIAN_POINT('Origin',(0.,-0.04763,0.));
#13681=CARTESIAN_POINT('',(-0.871530771444223,-0.04763,0.528110872004958));
#13682=CARTESIAN_POINT('Ctrl Pts',(-0.528110872004958,-0.0476300000000001,
0.871530771444223));
#13683=CARTESIAN_POINT('Ctrl Pts',(-0.530395067942936,-0.0609922781173484,
0.87014664509073));
#13684=CARTESIAN_POINT('Ctrl Pts',(-0.533674141594226,-0.0742967091364493,
0.868149331745851));
#13685=CARTESIAN_POINT('Ctrl Pts',(-0.54708917182331,-0.115492077056649,
0.85981294420286));
#13686=CARTESIAN_POINT('Ctrl Pts',(-0.560922177770136,-0.141695629206859,
0.850993704737257));
#13687=CARTESIAN_POINT('Ctrl Pts',(-0.590422647829571,-0.181890537957859,
0.830754510485543));
#13688=CARTESIAN_POINT('Ctrl Pts',(-0.609616703125488,-0.201072148666545,
0.816896541396381));
#13689=CARTESIAN_POINT('Ctrl Pts',(-0.641117951819998,-0.223955109275652,
0.792310597819928));
#13690=CARTESIAN_POINT('Ctrl Pts',(-0.657208095763053,-0.232742381310829,
0.779109323683611));
#13691=CARTESIAN_POINT('Ctrl Pts',(-0.68964083160521,-0.244234834628584,
0.750552691816205));
#13692=CARTESIAN_POINT('Ctrl Pts',(-0.705971972091755,-0.246942143572133,
0.735185187071673));
#13693=CARTESIAN_POINT('Ctrl Pts',(-0.735185187071673,-0.246942143572133,
0.705971972091754));
#13694=CARTESIAN_POINT('Ctrl Pts',(-0.750552691816206,-0.244234834628584,
0.689640831605209));
#13695=CARTESIAN_POINT('Ctrl Pts',(-0.779109323683612,-0.232742381310829,
0.657208095763052));
#13696=CARTESIAN_POINT('Ctrl Pts',(-0.792310597819928,-0.223955109275652,
0.641117951819998));
#13697=CARTESIAN_POINT('Ctrl Pts',(-0.816896541396382,-0.201072148666545,
0.609616703125487));
#13698=CARTESIAN_POINT('Ctrl Pts',(-0.830754510485544,-0.181890537957858,
0.590422647829571));
#13699=CARTESIAN_POINT('Ctrl Pts',(-0.850993704737257,-0.141695629206858,
0.560922177770135));
#13700=CARTESIAN_POINT('Ctrl Pts',(-0.859812944202861,-0.115492077056649,
0.547089171823309));
#13701=CARTESIAN_POINT('Ctrl Pts',(-0.868149331745852,-0.0742967091364491,
0.533674141594226));
#13702=CARTESIAN_POINT('Ctrl Pts',(-0.870146645090731,-0.0609922781173483,
0.530395067942936));
#13703=CARTESIAN_POINT('Ctrl Pts',(-0.871530771444223,-0.04763,0.528110872004958));
#13704=CARTESIAN_POINT('',(-0.989696097314,-0.04763,0.242834539687906));
#13705=CARTESIAN_POINT('Origin',(0.,-0.04763,0.));
#13706=CARTESIAN_POINT('',(-1.019052,-0.246942143572133,1.248489836334E-16));
#13707=CARTESIAN_POINT('Ctrl Pts',(-0.989696097314,-0.04763,0.242834539687906));
#13708=CARTESIAN_POINT('Ctrl Pts',(-0.990332542620729,-0.0609922781173483,
0.24024064412003));
#13709=CARTESIAN_POINT('Ctrl Pts',(-0.991238884025248,-0.0742967091364492,
0.236509675094874));
#13710=CARTESIAN_POINT('Ctrl Pts',(-0.994830026707808,-0.115492077056649,
0.221129100087819));
#13711=CARTESIAN_POINT('Ctrl Pts',(-0.998375294985966,-0.141695629206859,
0.205111543747588));
#13712=CARTESIAN_POINT('Ctrl Pts',(-1.00492400591205,-0.181890537957859,
0.169940289819232));
#13713=CARTESIAN_POINT('Ctrl Pts',(-1.00869718865384,-0.201072148666545,
0.1465689792446));
#13714=CARTESIAN_POINT('Ctrl Pts',(-1.01358704779679,-0.223955109275652,
0.106909345252088));
#13715=CARTESIAN_POINT('Ctrl Pts',(-1.0156297872271,-0.232742381310829,
0.0861971848975944));
#13716=CARTESIAN_POINT('Ctrl Pts',(-1.01837060663223,-0.244234834628584,
0.0430711894098825));
#13717=CARTESIAN_POINT('Ctrl Pts',(-1.019052,-0.246942143572133,0.0206568624125608));
#13718=CARTESIAN_POINT('Ctrl Pts',(-1.019052,-0.246942143572133,1.2490009027033E-16));
#13719=CARTESIAN_POINT('',(-1.019052,-0.28578,1.24797876996471E-16));
#13720=CARTESIAN_POINT('',(-1.019052,-0.166705,1.24797876996471E-16));
#13721=CARTESIAN_POINT('Origin',(0.,-0.28578,0.));
#13722=CARTESIAN_POINT('',(-0.989696097314,-0.04763,-0.242834539687906));
#13723=CARTESIAN_POINT('Ctrl Pts',(-1.019052,-0.246942143572133,1.2490009027033E-16));
#13724=CARTESIAN_POINT('Ctrl Pts',(-1.019052,-0.246942143572133,-0.0206568624125605));
#13725=CARTESIAN_POINT('Ctrl Pts',(-1.01837060663223,-0.244234834628584,
-0.0430711894098822));
#13726=CARTESIAN_POINT('Ctrl Pts',(-1.0156297872271,-0.232742381310829,
-0.0861971848975941));
#13727=CARTESIAN_POINT('Ctrl Pts',(-1.01358704779679,-0.223955109275652,
-0.106909345252087));
#13728=CARTESIAN_POINT('Ctrl Pts',(-1.00869718865384,-0.201072148666546,
-0.1465689792446));
#13729=CARTESIAN_POINT('Ctrl Pts',(-1.00492400591205,-0.181890537957859,
-0.169940289819232));
#13730=CARTESIAN_POINT('Ctrl Pts',(-0.998375294985966,-0.141695629206859,
-0.205111543747588));
#13731=CARTESIAN_POINT('Ctrl Pts',(-0.994830026707808,-0.11549207705665,
-0.221129100087819));
#13732=CARTESIAN_POINT('Ctrl Pts',(-0.991238884025248,-0.0742967091364495,
-0.236509675094874));
#13733=CARTESIAN_POINT('Ctrl Pts',(-0.990332542620729,-0.0609922781173484,
-0.24024064412003));
#13734=CARTESIAN_POINT('Ctrl Pts',(-0.989696097314,-0.0476300000000001,
-0.242834539687907));
#13735=CARTESIAN_POINT('',(-0.871530771444223,-0.04763,-0.528110872004958));
#13736=CARTESIAN_POINT('Origin',(0.,-0.04763,0.));
#13737=CARTESIAN_POINT('',(-0.528110872004958,-0.04763,-0.871530771444223));
#13738=CARTESIAN_POINT('Ctrl Pts',(-0.871530771444223,-0.0476300000000001,
-0.528110872004958));
#13739=CARTESIAN_POINT('Ctrl Pts',(-0.87014664509073,-0.0609922781173484,
-0.530395067942936));
#13740=CARTESIAN_POINT('Ctrl Pts',(-0.868149331745851,-0.0742967091364494,
-0.533674141594226));
#13741=CARTESIAN_POINT('Ctrl Pts',(-0.85981294420286,-0.115492077056649,
-0.54708917182331));
#13742=CARTESIAN_POINT('Ctrl Pts',(-0.850993704737257,-0.141695629206859,
-0.560922177770136));
#13743=CARTESIAN_POINT('Ctrl Pts',(-0.830754510485543,-0.181890537957859,
-0.590422647829571));
#13744=CARTESIAN_POINT('Ctrl Pts',(-0.816896541396381,-0.201072148666546,
-0.609616703125488));
#13745=CARTESIAN_POINT('Ctrl Pts',(-0.792310597819928,-0.223955109275652,
-0.641117951819999));
#13746=CARTESIAN_POINT('Ctrl Pts',(-0.779109323683611,-0.232742381310829,
-0.657208095763053));
#13747=CARTESIAN_POINT('Ctrl Pts',(-0.750552691816205,-0.244234834628584,
-0.68964083160521));
#13748=CARTESIAN_POINT('Ctrl Pts',(-0.735185187071673,-0.246942143572133,
-0.705971972091755));
#13749=CARTESIAN_POINT('Ctrl Pts',(-0.705971972091754,-0.246942143572133,
-0.735185187071673));
#13750=CARTESIAN_POINT('Ctrl Pts',(-0.68964083160521,-0.244234834628584,
-0.750552691816206));
#13751=CARTESIAN_POINT('Ctrl Pts',(-0.657208095763052,-0.232742381310829,
-0.779109323683612));
#13752=CARTESIAN_POINT('Ctrl Pts',(-0.641117951819998,-0.223955109275652,
-0.792310597819928));
#13753=CARTESIAN_POINT('Ctrl Pts',(-0.609616703125488,-0.201072148666545,
-0.816896541396381));
#13754=CARTESIAN_POINT('Ctrl Pts',(-0.590422647829571,-0.181890537957859,
-0.830754510485543));
#13755=CARTESIAN_POINT('Ctrl Pts',(-0.560922177770136,-0.141695629206859,
-0.850993704737257));
#13756=CARTESIAN_POINT('Ctrl Pts',(-0.54708917182331,-0.115492077056649,
-0.85981294420286));
#13757=CARTESIAN_POINT('Ctrl Pts',(-0.533674141594226,-0.0742967091364494,
-0.868149331745852));
#13758=CARTESIAN_POINT('Ctrl Pts',(-0.530395067942936,-0.0609922781173484,
-0.870146645090731));
#13759=CARTESIAN_POINT('Ctrl Pts',(-0.528110872004958,-0.0476300000000001,
-0.871530771444223));
#13760=CARTESIAN_POINT('',(-0.242834539687906,-0.04763,-0.989696097314));
#13761=CARTESIAN_POINT('Origin',(0.,-0.04763,0.));
#13762=CARTESIAN_POINT('',(0.242834539687906,-0.04763,-0.989696097314));
#13763=CARTESIAN_POINT('Ctrl Pts',(-0.242834539687907,-0.04763,-0.989696097314));
#13764=CARTESIAN_POINT('Ctrl Pts',(-0.24024064412003,-0.0609922781173483,
-0.990332542620729));
#13765=CARTESIAN_POINT('Ctrl Pts',(-0.236509675094874,-0.0742967091364493,
-0.991238884025248));
#13766=CARTESIAN_POINT('Ctrl Pts',(-0.221129100087819,-0.115492077056649,
-0.994830026707808));
#13767=CARTESIAN_POINT('Ctrl Pts',(-0.205111543747588,-0.141695629206859,
-0.998375294985966));
#13768=CARTESIAN_POINT('Ctrl Pts',(-0.169940289819232,-0.181890537957859,
-1.00492400591205));
#13769=CARTESIAN_POINT('Ctrl Pts',(-0.1465689792446,-0.201072148666545,
-1.00869718865384));
#13770=CARTESIAN_POINT('Ctrl Pts',(-0.106909345252087,-0.223955109275652,
-1.01358704779679));
#13771=CARTESIAN_POINT('Ctrl Pts',(-0.0861971848975942,-0.232742381310829,
-1.0156297872271));
#13772=CARTESIAN_POINT('Ctrl Pts',(-0.0430711894098823,-0.244234834628584,
-1.01837060663223));
#13773=CARTESIAN_POINT('Ctrl Pts',(-0.0206568624125606,-0.246942143572133,
-1.019052));
#13774=CARTESIAN_POINT('Ctrl Pts',(0.0206568624125607,-0.246942143572133,
-1.019052));
#13775=CARTESIAN_POINT('Ctrl Pts',(0.0430711894098824,-0.244234834628584,
-1.01837060663223));
#13776=CARTESIAN_POINT('Ctrl Pts',(0.0861971848975943,-0.232742381310829,
-1.0156297872271));
#13777=CARTESIAN_POINT('Ctrl Pts',(0.106909345252088,-0.223955109275652,
-1.01358704779679));
#13778=CARTESIAN_POINT('Ctrl Pts',(0.1465689792446,-0.201072148666545,-1.00869718865384));
#13779=CARTESIAN_POINT('Ctrl Pts',(0.169940289819232,-0.181890537957859,
-1.00492400591205));
#13780=CARTESIAN_POINT('Ctrl Pts',(0.205111543747588,-0.141695629206859,
-0.998375294985966));
#13781=CARTESIAN_POINT('Ctrl Pts',(0.221129100087819,-0.115492077056649,
-0.994830026707808));
#13782=CARTESIAN_POINT('Ctrl Pts',(0.236509675094874,-0.0742967091364493,
-0.991238884025248));
#13783=CARTESIAN_POINT('Ctrl Pts',(0.24024064412003,-0.0609922781173484,
-0.990332542620729));
#13784=CARTESIAN_POINT('Ctrl Pts',(0.242834539687907,-0.04763,-0.989696097314));
#13785=CARTESIAN_POINT('',(0.528110872004958,-0.04763,-0.871530771444223));
#13786=CARTESIAN_POINT('Origin',(0.,-0.04763,0.));
#13787=CARTESIAN_POINT('',(0.871530771444223,-0.04763,-0.528110872004958));
#13788=CARTESIAN_POINT('Ctrl Pts',(0.528110872004958,-0.0476300000000001,
-0.871530771444223));
#13789=CARTESIAN_POINT('Ctrl Pts',(0.530395067942936,-0.0609922781173484,
-0.870146645090731));
#13790=CARTESIAN_POINT('Ctrl Pts',(0.533674141594226,-0.0742967091364493,
-0.868149331745851));
#13791=CARTESIAN_POINT('Ctrl Pts',(0.54708917182331,-0.115492077056649,
-0.85981294420286));
#13792=CARTESIAN_POINT('Ctrl Pts',(0.560922177770136,-0.141695629206859,
-0.850993704737257));
#13793=CARTESIAN_POINT('Ctrl Pts',(0.590422647829571,-0.181890537957859,
-0.830754510485543));
#13794=CARTESIAN_POINT('Ctrl Pts',(0.609616703125488,-0.201072148666545,
-0.816896541396381));
#13795=CARTESIAN_POINT('Ctrl Pts',(0.641117951819998,-0.223955109275652,
-0.792310597819928));
#13796=CARTESIAN_POINT('Ctrl Pts',(0.657208095763053,-0.232742381310829,
-0.779109323683612));
#13797=CARTESIAN_POINT('Ctrl Pts',(0.68964083160521,-0.244234834628584,
-0.750552691816206));
#13798=CARTESIAN_POINT('Ctrl Pts',(0.705971972091755,-0.246942143572133,
-0.735185187071673));
#13799=CARTESIAN_POINT('Ctrl Pts',(0.735185187071673,-0.246942143572133,
-0.705971972091754));
#13800=CARTESIAN_POINT('Ctrl Pts',(0.750552691816206,-0.244234834628584,
-0.68964083160521));
#13801=CARTESIAN_POINT('Ctrl Pts',(0.779109323683612,-0.232742381310829,
-0.657208095763053));
#13802=CARTESIAN_POINT('Ctrl Pts',(0.792310597819928,-0.223955109275652,
-0.641117951819998));
#13803=CARTESIAN_POINT('Ctrl Pts',(0.816896541396381,-0.201072148666545,
-0.609616703125488));
#13804=CARTESIAN_POINT('Ctrl Pts',(0.830754510485543,-0.181890537957859,
-0.590422647829571));
#13805=CARTESIAN_POINT('Ctrl Pts',(0.850993704737257,-0.141695629206859,
-0.560922177770136));
#13806=CARTESIAN_POINT('Ctrl Pts',(0.85981294420286,-0.115492077056649,
-0.54708917182331));
#13807=CARTESIAN_POINT('Ctrl Pts',(0.868149331745851,-0.0742967091364493,
-0.533674141594226));
#13808=CARTESIAN_POINT('Ctrl Pts',(0.870146645090731,-0.0609922781173484,
-0.530395067942936));
#13809=CARTESIAN_POINT('Ctrl Pts',(0.871530771444223,-0.0476300000000001,
-0.528110872004958));
#13810=CARTESIAN_POINT('',(0.989696097314,-0.04763,-0.242834539687906));
#13811=CARTESIAN_POINT('Origin',(0.,-0.04763,0.));
#13812=CARTESIAN_POINT('',(0.989696097314,-0.04763,0.242834539687906));
#13813=CARTESIAN_POINT('Ctrl Pts',(0.989696097314,-0.04763,-0.242834539687907));
#13814=CARTESIAN_POINT('Ctrl Pts',(0.990332542620729,-0.0609922781173483,
-0.24024064412003));
#13815=CARTESIAN_POINT('Ctrl Pts',(0.991238884025248,-0.0742967091364493,
-0.236509675094874));
#13816=CARTESIAN_POINT('Ctrl Pts',(0.994830026707808,-0.115492077056649,
-0.221129100087819));
#13817=CARTESIAN_POINT('Ctrl Pts',(0.998375294985966,-0.141695629206859,
-0.205111543747588));
#13818=CARTESIAN_POINT('Ctrl Pts',(1.00492400591205,-0.181890537957859,
-0.169940289819232));
#13819=CARTESIAN_POINT('Ctrl Pts',(1.00869718865384,-0.201072148666545,
-0.1465689792446));
#13820=CARTESIAN_POINT('Ctrl Pts',(1.01358704779679,-0.223955109275652,
-0.106909345252087));
#13821=CARTESIAN_POINT('Ctrl Pts',(1.0156297872271,-0.232742381310829,-0.0861971848975942));
#13822=CARTESIAN_POINT('Ctrl Pts',(1.01837060663223,-0.244234834628584,
-0.0430711894098823));
#13823=CARTESIAN_POINT('Ctrl Pts',(1.019052,-0.246942143572133,-0.0206568624125607));
#13824=CARTESIAN_POINT('Ctrl Pts',(1.019052,-0.246942143572133,0.0206568624125607));
#13825=CARTESIAN_POINT('Ctrl Pts',(1.01837060663223,-0.244234834628584,
0.0430711894098823));
#13826=CARTESIAN_POINT('Ctrl Pts',(1.0156297872271,-0.232742381310829,0.0861971848975942));
#13827=CARTESIAN_POINT('Ctrl Pts',(1.01358704779679,-0.223955109275652,
0.106909345252087));
#13828=CARTESIAN_POINT('Ctrl Pts',(1.00869718865384,-0.201072148666545,
0.1465689792446));
#13829=CARTESIAN_POINT('Ctrl Pts',(1.00492400591205,-0.181890537957859,
0.169940289819232));
#13830=CARTESIAN_POINT('Ctrl Pts',(0.998375294985966,-0.141695629206859,
0.205111543747588));
#13831=CARTESIAN_POINT('Ctrl Pts',(0.994830026707808,-0.115492077056649,
0.221129100087819));
#13832=CARTESIAN_POINT('Ctrl Pts',(0.991238884025248,-0.0742967091364492,
0.236509675094874));
#13833=CARTESIAN_POINT('Ctrl Pts',(0.990332542620729,-0.0609922781173483,
0.24024064412003));
#13834=CARTESIAN_POINT('Ctrl Pts',(0.989696097314,-0.04763,0.242834539687907));
#13835=CARTESIAN_POINT('Origin',(0.,-0.04763,0.));
#13836=CARTESIAN_POINT('Origin',(0.,-0.04763,0.));
#13837=CARTESIAN_POINT('',(0.238183666596899,-0.04763,0.951592097314));
#13838=CARTESIAN_POINT('Origin',(0.,-0.04763,0.));
#13839=CARTESIAN_POINT('Origin',(-1.94289029309402E-16,-0.04763,1.));
#13840=CARTESIAN_POINT('Origin',(-1.94289029309402E-16,0.,1.));
#13841=CARTESIAN_POINT('',(-0.2381836665969,-0.04763,0.951592097314));
#13842=CARTESIAN_POINT('Ctrl Pts',(-0.238183666596899,-0.0476299999999999,
0.951592097314));
#13843=CARTESIAN_POINT('Ctrl Pts',(-0.233157223576062,-0.0740444353928835,
0.952850216871763));
#13844=CARTESIAN_POINT('Ctrl Pts',(-0.223801617934946,-0.0999305678883309,
0.955173119738174));
#13845=CARTESIAN_POINT('Ctrl Pts',(-0.199966927975188,-0.142345102874864,
0.960411259488514));
#13846=CARTESIAN_POINT('Ctrl Pts',(-0.1868781821531,-0.159766064500479,
0.963103647174702));
#13847=CARTESIAN_POINT('Ctrl Pts',(-0.15681442133453,-0.190326085855194,
0.968453058988463));
#13848=CARTESIAN_POINT('Ctrl Pts',(-0.139836317888043,-0.203463743702801,
0.971100730005489));
#13849=CARTESIAN_POINT('Ctrl Pts',(-0.104422493053067,-0.224161999508995,
0.975530745318961));
#13850=CARTESIAN_POINT('Ctrl Pts',(-0.0842175114474176,-0.232861760990032,
0.977553872336861));
#13851=CARTESIAN_POINT('Ctrl Pts',(-0.0421062857595701,-0.244251601209411,
0.980270995488453));
#13852=CARTESIAN_POINT('Ctrl Pts',(-0.0201990724523197,-0.246942143572133,
0.980948));
#13853=CARTESIAN_POINT('Ctrl Pts',(0.020199072452319,-0.246942143572133,
0.980948));
#13854=CARTESIAN_POINT('Ctrl Pts',(0.0421062857595694,-0.244251601209411,
0.980270995488454));
#13855=CARTESIAN_POINT('Ctrl Pts',(0.0842175114474169,-0.232861760990032,
0.977553872336861));
#13856=CARTESIAN_POINT('Ctrl Pts',(0.104422493053067,-0.224161999508995,
0.975530745318961));
#13857=CARTESIAN_POINT('Ctrl Pts',(0.139836317888042,-0.203463743702801,
0.971100730005489));
#13858=CARTESIAN_POINT('Ctrl Pts',(0.15681442133453,-0.190326085855194,
0.968453058988463));
#13859=CARTESIAN_POINT('Ctrl Pts',(0.1868781821531,-0.15976606450048,0.963103647174702));
#13860=CARTESIAN_POINT('Ctrl Pts',(0.199966927975188,-0.142345102874864,
0.960411259488514));
#13861=CARTESIAN_POINT('Ctrl Pts',(0.223801617934945,-0.0999305678883309,
0.955173119738174));
#13862=CARTESIAN_POINT('Ctrl Pts',(0.233157223576061,-0.0740444353928835,
0.952850216871763));
#13863=CARTESIAN_POINT('Ctrl Pts',(0.238183666596899,-0.0476299999999999,
0.951592097314));
#13864=CARTESIAN_POINT('Origin',(-1.94289029309402E-16,-0.04763,1.));
#13865=CARTESIAN_POINT('Origin',(0.,-0.04763,0.));
#13866=CARTESIAN_POINT('',(-0.504455939115715,-0.04763,0.841298510752802));
#13867=CARTESIAN_POINT('Origin',(0.,-0.04763,0.));
#13868=CARTESIAN_POINT('Origin',(-0.707106781186548,-0.04763,0.707106781186547));
#13869=CARTESIAN_POINT('Origin',(-0.707106781186548,0.,0.707106781186547));
#13870=CARTESIAN_POINT('',(-0.841298510752802,-0.04763,0.504455939115715));
#13871=CARTESIAN_POINT('Ctrl Pts',(-0.841298510752802,-0.04763,0.504455939115715));
#13872=CARTESIAN_POINT('Ctrl Pts',(-0.838633903678357,-0.0740444353928835,
0.508899795931835));
#13873=CARTESIAN_POINT('Ctrl Pts',(-0.833661031856294,-0.0999305678883309,
0.517157748491652));
#13874=CARTESIAN_POINT('Ctrl Pts',(-0.820511285096538,-0.142345102874864,
0.537715343527944));
#13875=CARTESIAN_POINT('Ctrl Pts',(-0.813159949759,-0.159766064500479,0.548874290046456));
#13876=CARTESIAN_POINT('Ctrl Pts',(-0.795684265985089,-0.190326085855194,
0.573915184558107));
#13877=CARTESIAN_POINT('Ctrl Pts',(-0.78555112003688,-0.203463743702801,
0.587792702767295));
#13878=CARTESIAN_POINT('Ctrl Pts',(-0.763642258217233,-0.224161999508995,
0.615966552324775));
#13879=CARTESIAN_POINT('Ctrl Pts',(-0.750785745543687,-0.232861760990032,
0.631684198665438));
#13880=CARTESIAN_POINT('Ctrl Pts',(-0.722929908501543,-0.244251601209411,
0.663382628119203));
#13881=CARTESIAN_POINT('Ctrl Pts',(-0.707917883896095,-0.246942143572133,
0.679352081686668));
#13882=CARTESIAN_POINT('Ctrl Pts',(-0.679352081686668,-0.246942143572133,
0.707917883896095));
#13883=CARTESIAN_POINT('Ctrl Pts',(-0.663382628119203,-0.244251601209411,
0.722929908501544));
#13884=CARTESIAN_POINT('Ctrl Pts',(-0.631684198665438,-0.232861760990031,
0.750785745543687));
#13885=CARTESIAN_POINT('Ctrl Pts',(-0.615966552324775,-0.224161999508995,
0.763642258217233));
#13886=CARTESIAN_POINT('Ctrl Pts',(-0.587792702767295,-0.203463743702801,
0.78555112003688));
#13887=CARTESIAN_POINT('Ctrl Pts',(-0.573915184558107,-0.190326085855194,
0.795684265985088));
#13888=CARTESIAN_POINT('Ctrl Pts',(-0.548874290046456,-0.159766064500479,
0.813159949759));
#13889=CARTESIAN_POINT('Ctrl Pts',(-0.537715343527944,-0.142345102874864,
0.820511285096538));
#13890=CARTESIAN_POINT('Ctrl Pts',(-0.517157748491652,-0.0999305678883309,
0.833661031856294));
#13891=CARTESIAN_POINT('Ctrl Pts',(-0.508899795931835,-0.0740444353928835,
0.838633903678357));
#13892=CARTESIAN_POINT('Ctrl Pts',(-0.504455939115716,-0.04763,0.841298510752801));
#13893=CARTESIAN_POINT('Origin',(-0.707106781186548,-0.04763,0.707106781186547));
#13894=CARTESIAN_POINT('Origin',(0.,-0.04763,0.));
#13895=CARTESIAN_POINT('',(-0.951592097314,-0.04763,0.238183666596899));
#13896=CARTESIAN_POINT('Origin',(0.,-0.04763,0.));
#13897=CARTESIAN_POINT('Origin',(-1.,-0.04763,-1.11022302462516E-16));
#13898=CARTESIAN_POINT('Origin',(-1.,0.,-1.11022302462516E-16));
#13899=CARTESIAN_POINT('',(-0.951592097314,-0.04763,-0.2381836665969));
#13900=CARTESIAN_POINT('',(-0.980948,-0.246942143572133,1.08514323328844E-18));
#13901=CARTESIAN_POINT('Ctrl Pts',(-0.951592097314,-0.04763,-0.238183666596899));
#13902=CARTESIAN_POINT('Ctrl Pts',(-0.952850216871763,-0.0740444353928835,
-0.233157223576062));
#13903=CARTESIAN_POINT('Ctrl Pts',(-0.955173119738174,-0.0999305678883309,
-0.223801617934946));
#13904=CARTESIAN_POINT('Ctrl Pts',(-0.960411259488514,-0.142345102874864,
-0.199966927975188));
#13905=CARTESIAN_POINT('Ctrl Pts',(-0.963103647174702,-0.159766064500479,
-0.1868781821531));
#13906=CARTESIAN_POINT('Ctrl Pts',(-0.968453058988463,-0.190326085855194,
-0.15681442133453));
#13907=CARTESIAN_POINT('Ctrl Pts',(-0.971100730005489,-0.203463743702801,
-0.139836317888043));
#13908=CARTESIAN_POINT('Ctrl Pts',(-0.975530745318961,-0.224161999508995,
-0.104422493053067));
#13909=CARTESIAN_POINT('Ctrl Pts',(-0.977553872336861,-0.232861760990032,
-0.0842175114474175));
#13910=CARTESIAN_POINT('Ctrl Pts',(-0.980270995488453,-0.244251601209411,
-0.0421062857595699));
#13911=CARTESIAN_POINT('Ctrl Pts',(-0.980948,-0.246942143572133,-0.0201990724523195));
#13912=CARTESIAN_POINT('Ctrl Pts',(-0.980948,-0.246942143572133,-1.17961196366423E-16));
#13913=CARTESIAN_POINT('Origin',(-1.,-0.04763,-1.11022302462516E-16));
#13914=CARTESIAN_POINT('Ctrl Pts',(-0.980948,-0.246942143572133,-1.17961196366423E-16));
#13915=CARTESIAN_POINT('Ctrl Pts',(-0.980948,-0.246942143572133,0.0201990724523192));
#13916=CARTESIAN_POINT('Ctrl Pts',(-0.980270995488453,-0.244251601209411,
0.0421062857595695));
#13917=CARTESIAN_POINT('Ctrl Pts',(-0.977553872336861,-0.232861760990032,
0.0842175114474169));
#13918=CARTESIAN_POINT('Ctrl Pts',(-0.975530745318961,-0.224161999508995,
0.104422493053066));
#13919=CARTESIAN_POINT('Ctrl Pts',(-0.971100730005489,-0.203463743702801,
0.139836317888042));
#13920=CARTESIAN_POINT('Ctrl Pts',(-0.968453058988463,-0.190326085855194,
0.15681442133453));
#13921=CARTESIAN_POINT('Ctrl Pts',(-0.963103647174702,-0.15976606450048,
0.1868781821531));
#13922=CARTESIAN_POINT('Ctrl Pts',(-0.960411259488514,-0.142345102874864,
0.199966927975188));
#13923=CARTESIAN_POINT('Ctrl Pts',(-0.955173119738174,-0.099930567888331,
0.223801617934945));
#13924=CARTESIAN_POINT('Ctrl Pts',(-0.952850216871763,-0.0740444353928835,
0.233157223576061));
#13925=CARTESIAN_POINT('Ctrl Pts',(-0.951592097314,-0.04763,0.238183666596899));
#13926=CARTESIAN_POINT('Origin',(0.,-0.04763,0.));
#13927=CARTESIAN_POINT('',(-0.841298510752802,-0.04763,-0.504455939115715));
#13928=CARTESIAN_POINT('Origin',(0.,-0.04763,0.));
#13929=CARTESIAN_POINT('Origin',(-0.707106781186547,-0.04763,-0.707106781186548));
#13930=CARTESIAN_POINT('Origin',(-0.707106781186547,0.,-0.707106781186548));
#13931=CARTESIAN_POINT('',(-0.504455939115715,-0.04763,-0.841298510752802));
#13932=CARTESIAN_POINT('Ctrl Pts',(-0.504455939115715,-0.04763,-0.841298510752802));
#13933=CARTESIAN_POINT('Ctrl Pts',(-0.508899795931835,-0.0740444353928835,
-0.838633903678357));
#13934=CARTESIAN_POINT('Ctrl Pts',(-0.517157748491652,-0.0999305678883309,
-0.833661031856294));
#13935=CARTESIAN_POINT('Ctrl Pts',(-0.537715343527944,-0.142345102874864,
-0.820511285096538));
#13936=CARTESIAN_POINT('Ctrl Pts',(-0.548874290046456,-0.159766064500479,
-0.813159949759));
#13937=CARTESIAN_POINT('Ctrl Pts',(-0.573915184558107,-0.190326085855194,
-0.795684265985089));
#13938=CARTESIAN_POINT('Ctrl Pts',(-0.587792702767295,-0.203463743702801,
-0.78555112003688));
#13939=CARTESIAN_POINT('Ctrl Pts',(-0.615966552324775,-0.224161999508995,
-0.763642258217233));
#13940=CARTESIAN_POINT('Ctrl Pts',(-0.631684198665438,-0.232861760990032,
-0.750785745543687));
#13941=CARTESIAN_POINT('Ctrl Pts',(-0.663382628119203,-0.244251601209411,
-0.722929908501543));
#13942=CARTESIAN_POINT('Ctrl Pts',(-0.679352081686668,-0.246942143572133,
-0.707917883896095));
#13943=CARTESIAN_POINT('Ctrl Pts',(-0.707917883896095,-0.246942143572133,
-0.679352081686668));
#13944=CARTESIAN_POINT('Ctrl Pts',(-0.722929908501543,-0.244251601209411,
-0.663382628119203));
#13945=CARTESIAN_POINT('Ctrl Pts',(-0.750785745543687,-0.232861760990032,
-0.631684198665439));
#13946=CARTESIAN_POINT('Ctrl Pts',(-0.763642258217232,-0.224161999508995,
-0.615966552324775));
#13947=CARTESIAN_POINT('Ctrl Pts',(-0.78555112003688,-0.203463743702801,
-0.587792702767295));
#13948=CARTESIAN_POINT('Ctrl Pts',(-0.795684265985088,-0.190326085855194,
-0.573915184558107));
#13949=CARTESIAN_POINT('Ctrl Pts',(-0.813159949759,-0.15976606450048,-0.548874290046456));
#13950=CARTESIAN_POINT('Ctrl Pts',(-0.820511285096538,-0.142345102874864,
-0.537715343527944));
#13951=CARTESIAN_POINT('Ctrl Pts',(-0.833661031856294,-0.0999305678883311,
-0.517157748491652));
#13952=CARTESIAN_POINT('Ctrl Pts',(-0.838633903678357,-0.0740444353928836,
-0.508899795931835));
#13953=CARTESIAN_POINT('Ctrl Pts',(-0.841298510752801,-0.04763,-0.504455939115715));
#13954=CARTESIAN_POINT('Origin',(-0.707106781186547,-0.04763,-0.707106781186548));
#13955=CARTESIAN_POINT('Origin',(0.,-0.04763,0.));
#13956=CARTESIAN_POINT('',(-0.238183666596899,-0.04763,-0.951592097314));
#13957=CARTESIAN_POINT('Origin',(0.,-0.04763,0.));
#13958=CARTESIAN_POINT('Origin',(5.55111512312578E-17,-0.04763,-1.));
#13959=CARTESIAN_POINT('Origin',(5.55111512312578E-17,0.,-1.));
#13960=CARTESIAN_POINT('',(0.238183666596899,-0.04763,-0.951592097314));
#13961=CARTESIAN_POINT('Ctrl Pts',(0.238183666596899,-0.04763,-0.951592097314));
#13962=CARTESIAN_POINT('Ctrl Pts',(0.233157223576062,-0.0740444353928835,
-0.952850216871763));
#13963=CARTESIAN_POINT('Ctrl Pts',(0.223801617934946,-0.099930567888331,
-0.955173119738174));
#13964=CARTESIAN_POINT('Ctrl Pts',(0.199966927975188,-0.142345102874864,
-0.960411259488514));
#13965=CARTESIAN_POINT('Ctrl Pts',(0.1868781821531,-0.15976606450048,-0.963103647174702));
#13966=CARTESIAN_POINT('Ctrl Pts',(0.15681442133453,-0.190326085855194,
-0.968453058988463));
#13967=CARTESIAN_POINT('Ctrl Pts',(0.139836317888042,-0.203463743702801,
-0.971100730005489));
#13968=CARTESIAN_POINT('Ctrl Pts',(0.104422493053067,-0.224161999508995,
-0.975530745318961));
#13969=CARTESIAN_POINT('Ctrl Pts',(0.0842175114474173,-0.232861760990032,
-0.977553872336861));
#13970=CARTESIAN_POINT('Ctrl Pts',(0.0421062857595698,-0.244251601209411,
-0.980270995488453));
#13971=CARTESIAN_POINT('Ctrl Pts',(0.0201990724523194,-0.246942143572133,
-0.980948));
#13972=CARTESIAN_POINT('Ctrl Pts',(-0.0201990724523193,-0.246942143572133,
-0.980948));
#13973=CARTESIAN_POINT('Ctrl Pts',(-0.0421062857595697,-0.244251601209411,
-0.980270995488453));
#13974=CARTESIAN_POINT('Ctrl Pts',(-0.0842175114474171,-0.232861760990032,
-0.977553872336861));
#13975=CARTESIAN_POINT('Ctrl Pts',(-0.104422493053067,-0.224161999508995,
-0.975530745318961));
#13976=CARTESIAN_POINT('Ctrl Pts',(-0.139836317888042,-0.203463743702801,
-0.971100730005489));
#13977=CARTESIAN_POINT('Ctrl Pts',(-0.15681442133453,-0.190326085855194,
-0.968453058988463));
#13978=CARTESIAN_POINT('Ctrl Pts',(-0.1868781821531,-0.15976606450048,-0.963103647174702));
#13979=CARTESIAN_POINT('Ctrl Pts',(-0.199966927975188,-0.142345102874864,
-0.960411259488514));
#13980=CARTESIAN_POINT('Ctrl Pts',(-0.223801617934945,-0.099930567888331,
-0.955173119738174));
#13981=CARTESIAN_POINT('Ctrl Pts',(-0.233157223576062,-0.0740444353928835,
-0.952850216871763));
#13982=CARTESIAN_POINT('Ctrl Pts',(-0.238183666596899,-0.0476299999999999,
-0.951592097314));
#13983=CARTESIAN_POINT('Origin',(5.55111512312578E-17,-0.04763,-1.));
#13984=CARTESIAN_POINT('Origin',(0.,-0.04763,0.));
#13985=CARTESIAN_POINT('',(0.504455939115715,-0.04763,-0.841298510752802));
#13986=CARTESIAN_POINT('Origin',(0.,-0.04763,0.));
#13987=CARTESIAN_POINT('Origin',(0.707106781186548,-0.04763,-0.707106781186547));
#13988=CARTESIAN_POINT('Origin',(0.707106781186548,0.,-0.707106781186547));
#13989=CARTESIAN_POINT('',(0.841298510752802,-0.04763,-0.504455939115715));
#13990=CARTESIAN_POINT('Ctrl Pts',(0.841298510752802,-0.04763,-0.504455939115715));
#13991=CARTESIAN_POINT('Ctrl Pts',(0.838633903678357,-0.0740444353928835,
-0.508899795931835));
#13992=CARTESIAN_POINT('Ctrl Pts',(0.833661031856294,-0.0999305678883309,
-0.517157748491652));
#13993=CARTESIAN_POINT('Ctrl Pts',(0.820511285096538,-0.142345102874864,
-0.537715343527944));
#13994=CARTESIAN_POINT('Ctrl Pts',(0.813159949759,-0.159766064500479,-0.548874290046456));
#13995=CARTESIAN_POINT('Ctrl Pts',(0.795684265985088,-0.190326085855194,
-0.573915184558107));
#13996=CARTESIAN_POINT('Ctrl Pts',(0.78555112003688,-0.203463743702801,
-0.587792702767295));
#13997=CARTESIAN_POINT('Ctrl Pts',(0.763642258217233,-0.224161999508995,
-0.615966552324775));
#13998=CARTESIAN_POINT('Ctrl Pts',(0.750785745543687,-0.232861760990032,
-0.631684198665438));
#13999=CARTESIAN_POINT('Ctrl Pts',(0.722929908501543,-0.244251601209411,
-0.663382628119203));
#14000=CARTESIAN_POINT('Ctrl Pts',(0.707917883896095,-0.246942143572133,
-0.679352081686668));
#14001=CARTESIAN_POINT('Ctrl Pts',(0.679352081686668,-0.246942143572133,
-0.707917883896095));
#14002=CARTESIAN_POINT('Ctrl Pts',(0.663382628119203,-0.244251601209411,
-0.722929908501543));
#14003=CARTESIAN_POINT('Ctrl Pts',(0.631684198665438,-0.232861760990032,
-0.750785745543687));
#14004=CARTESIAN_POINT('Ctrl Pts',(0.615966552324775,-0.224161999508995,
-0.763642258217232));
#14005=CARTESIAN_POINT('Ctrl Pts',(0.587792702767295,-0.203463743702801,
-0.78555112003688));
#14006=CARTESIAN_POINT('Ctrl Pts',(0.573915184558107,-0.190326085855194,
-0.795684265985088));
#14007=CARTESIAN_POINT('Ctrl Pts',(0.548874290046456,-0.159766064500479,
-0.813159949759));
#14008=CARTESIAN_POINT('Ctrl Pts',(0.537715343527944,-0.142345102874864,
-0.820511285096538));
#14009=CARTESIAN_POINT('Ctrl Pts',(0.517157748491652,-0.099930567888331,
-0.833661031856294));
#14010=CARTESIAN_POINT('Ctrl Pts',(0.508899795931835,-0.0740444353928835,
-0.838633903678357));
#14011=CARTESIAN_POINT('Ctrl Pts',(0.504455939115715,-0.04763,-0.841298510752801));
#14012=CARTESIAN_POINT('Origin',(0.707106781186548,-0.04763,-0.707106781186547));
#14013=CARTESIAN_POINT('Origin',(0.,-0.166705,0.));
#14014=CARTESIAN_POINT('',(-0.980948,-0.28578,1.20131482833E-16));
#14015=CARTESIAN_POINT('Origin',(0.,-0.28578,0.));
#14016=CARTESIAN_POINT('',(-0.980948,-0.166705,1.20131482833E-16));
#14017=CARTESIAN_POINT('',(0.951592097314,-0.04763,0.238183666596899));
#14018=CARTESIAN_POINT('Origin',(0.,-0.04763,0.));
#14019=CARTESIAN_POINT('',(0.951592097314,-0.04763,-0.238183666596899));
#14020=CARTESIAN_POINT('Ctrl Pts',(0.951592097314,-0.04763,0.238183666596899));
#14021=CARTESIAN_POINT('Ctrl Pts',(0.952850216871763,-0.0740444353928835,
0.233157223576062));
#14022=CARTESIAN_POINT('Ctrl Pts',(0.955173119738174,-0.099930567888331,
0.223801617934945));
#14023=CARTESIAN_POINT('Ctrl Pts',(0.960411259488514,-0.142345102874864,
0.199966927975188));
#14024=CARTESIAN_POINT('Ctrl Pts',(0.963103647174702,-0.15976606450048,
0.1868781821531));
#14025=CARTESIAN_POINT('Ctrl Pts',(0.968453058988463,-0.190326085855194,
0.15681442133453));
#14026=CARTESIAN_POINT('Ctrl Pts',(0.971100730005489,-0.203463743702801,
0.139836317888042));
#14027=CARTESIAN_POINT('Ctrl Pts',(0.975530745318961,-0.224161999508995,
0.104422493053067));
#14028=CARTESIAN_POINT('Ctrl Pts',(0.977553872336861,-0.232861760990032,
0.0842175114474172));
#14029=CARTESIAN_POINT('Ctrl Pts',(0.980270995488453,-0.244251601209411,
0.0421062857595697));
#14030=CARTESIAN_POINT('Ctrl Pts',(0.980948,-0.246942143572133,0.0201990724523194));
#14031=CARTESIAN_POINT('Ctrl Pts',(0.980948,-0.246942143572133,-0.0201990724523194));
#14032=CARTESIAN_POINT('Ctrl Pts',(0.980270995488453,-0.244251601209411,
-0.0421062857595697));
#14033=CARTESIAN_POINT('Ctrl Pts',(0.977553872336861,-0.232861760990032,
-0.0842175114474172));
#14034=CARTESIAN_POINT('Ctrl Pts',(0.975530745318961,-0.224161999508995,
-0.104422493053067));
#14035=CARTESIAN_POINT('Ctrl Pts',(0.971100730005489,-0.203463743702801,
-0.139836317888042));
#14036=CARTESIAN_POINT('Ctrl Pts',(0.968453058988463,-0.190326085855194,
-0.15681442133453));
#14037=CARTESIAN_POINT('Ctrl Pts',(0.963103647174702,-0.15976606450048,
-0.1868781821531));
#14038=CARTESIAN_POINT('Ctrl Pts',(0.960411259488514,-0.142345102874864,
-0.199966927975188));
#14039=CARTESIAN_POINT('Ctrl Pts',(0.955173119738174,-0.099930567888331,
-0.223801617934945));
#14040=CARTESIAN_POINT('Ctrl Pts',(0.952850216871763,-0.0740444353928835,
-0.233157223576062));
#14041=CARTESIAN_POINT('Ctrl Pts',(0.951592097314,-0.0476299999999999,-0.238183666596899));
#14042=CARTESIAN_POINT('Origin',(0.,-0.04763,0.));
#14043=CARTESIAN_POINT('Origin',(0.,-0.04763,0.));
#14044=CARTESIAN_POINT('Origin',(1.,-0.04763,0.));
#14045=CARTESIAN_POINT('Origin',(1.,0.,0.));
#14046=CARTESIAN_POINT('Origin',(1.,-0.04763,0.));
#14047=CARTESIAN_POINT('Origin',(0.,-0.28578,0.));
#14048=CARTESIAN_POINT('Origin',(0.,-0.04763,0.));
#15135=UNCERTAINTY_MEASURE_WITH_UNIT(LENGTH_MEASURE(0.001),#15213,
'DISTANCE_ACCURACY_VALUE',
'Maximum model space distance between geometric entities at asserted c
onnectivities');
#15162=UNCERTAINTY_MEASURE_WITH_UNIT(LENGTH_MEASURE(0.001),#15213,
'DISTANCE_ACCURACY_VALUE',
'Maximum model space distance between geometric entities at asserted c
onnectivities');
#15185=(
GEOMETRIC_REPRESENTATION_CONTEXT(3)
GLOBAL_UNCERTAINTY_ASSIGNED_CONTEXT((#15135))
GLOBAL_UNIT_ASSIGNED_CONTEXT((#15213,#15215,#15216))
REPRESENTATION_CONTEXT('','3D')
);
#15212=(
GEOMETRIC_REPRESENTATION_CONTEXT(3)
GLOBAL_UNCERTAINTY_ASSIGNED_CONTEXT((#15162))
GLOBAL_UNIT_ASSIGNED_CONTEXT((#15213,#15215,#15216))
REPRESENTATION_CONTEXT('','3D')
);
#15213=(
LENGTH_UNIT()
NAMED_UNIT(*)
SI_UNIT(.CENTI.,.METRE.)
);
#15215=(
NAMED_UNIT(*)
PLANE_ANGLE_UNIT()
SI_UNIT($,.RADIAN.)
);
#15216=(
NAMED_UNIT(*)
SI_UNIT($,.STERADIAN.)
SOLID_ANGLE_UNIT()
);
#15239=SHAPE_DEFINITION_REPRESENTATION(#15288,#15423);
#15288=PRODUCT_DEFINITION_SHAPE('',$,#15473);
#15423=SHAPE_REPRESENTATION('',(#9222),#15185);
#15450=PRODUCT_DEFINITION_CONTEXT('part definition',#15599,'design');
#15473=PRODUCT_DEFINITION('Cage','Cage',#15522,#15450);
#15522=PRODUCT_DEFINITION_FORMATION('',$,#15623);
#15599=APPLICATION_CONTEXT(
'Core Data for Automotive Mechanical Design Process');
#15600=PRODUCT_CONTEXT('part definition',#15599,'mechanical');
#15623=PRODUCT('Cage','Cage','Cage',(#15600));
#15713=COLOUR_RGB('Grey',0.48,0.52,0.57);
#15714=FILL_AREA_STYLE_COLOUR('',#15713);
#15715=FILL_AREA_STYLE('',(#15714));
#15716=SURFACE_STYLE_FILL_AREA(#15715);
#15717=SURFACE_SIDE_STYLE('',(#15716));
#15718=SURFACE_STYLE_USAGE(.BOTH.,#15717);
#15719=PRESENTATION_STYLE_ASSIGNMENT((#15718));
ENDSEC;
END-ISO-10303-21;
